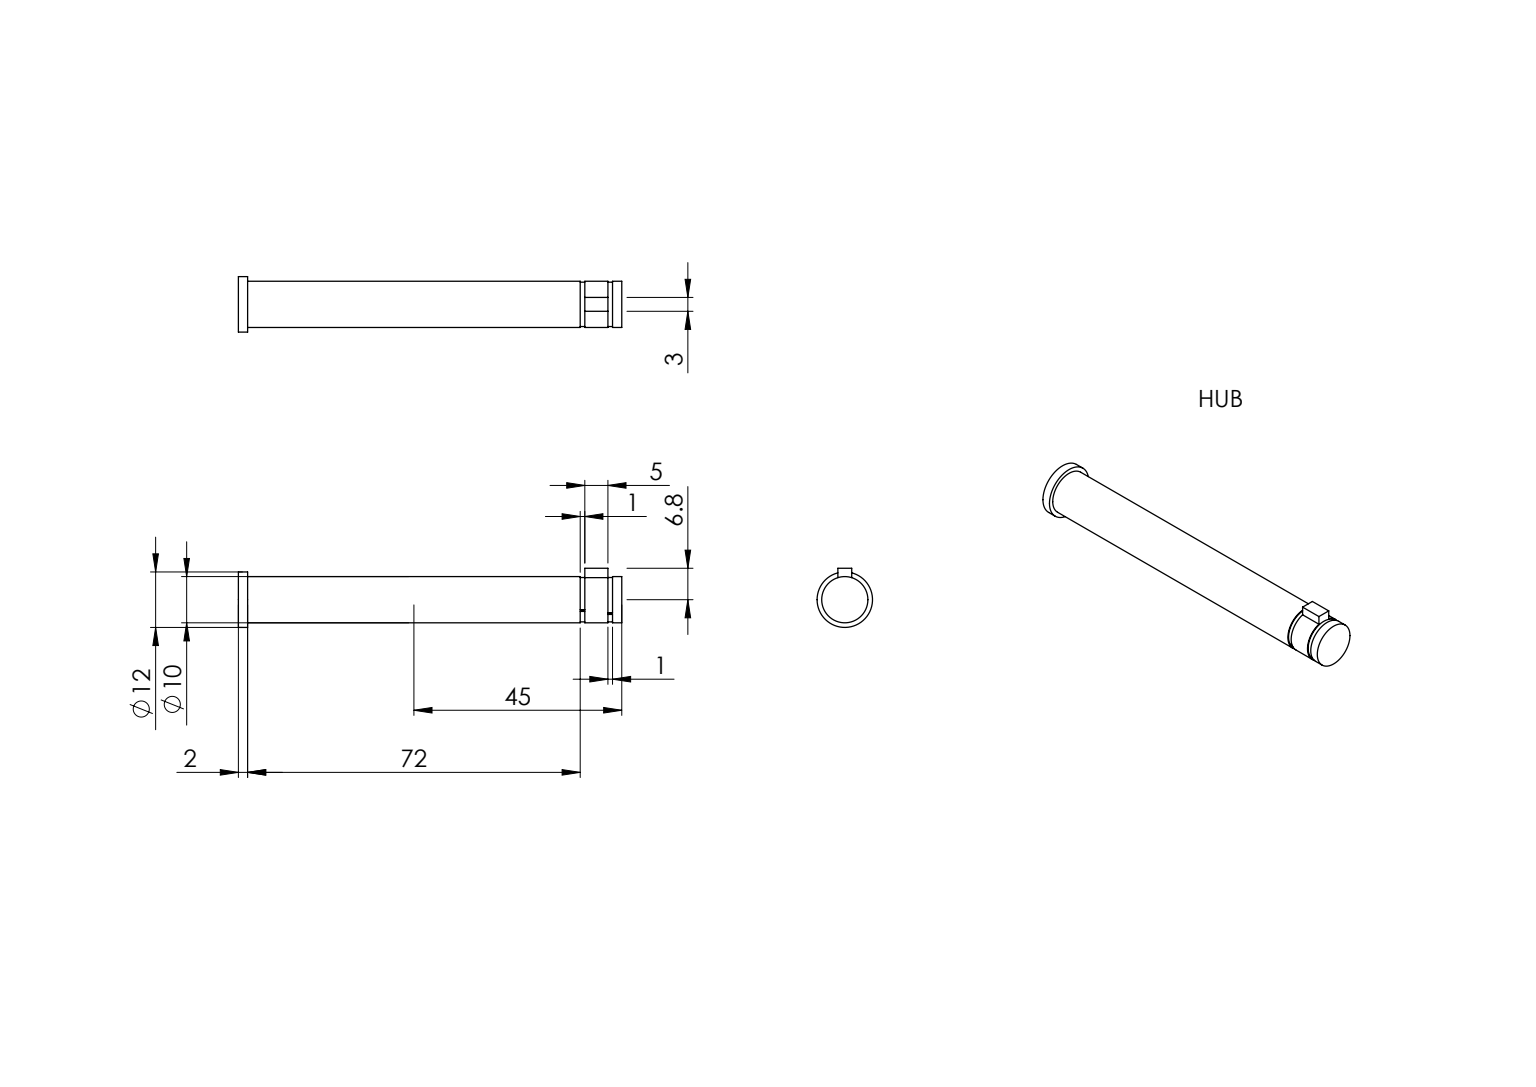
ISO-10303-21;
HEADER;
FILE_DESCRIPTION (('STEP AP214'),
    '1' );
FILE_NAME ('hub.step',
    '2026-10-27T08:02:39',
    ( '' ),
    ( '' ),
    'SwSTEP 2.0',
    'SolidWorks 2026',
    '' );
FILE_SCHEMA (( 'AUTOMOTIVE_DESIGN' ));
ENDSEC;

DATA;
#62=VECTOR ( 'NONE', #7382, 1000.000000000000000 ) ;
#68=DIRECTION ( 'NONE',  ( -1.000000000000000000, -3.903127820947815962E-18, 0.000000000000000000 ) ) ;
#73=CARTESIAN_POINT ( 'NONE',  ( 37.00000000000000711, 6.799999999999998046, 1.500000000000000000 ) ) ;
#88=VERTEX_POINT ( 'NONE', #10671 ) ;
#155=SHAPE_DEFINITION_REPRESENTATION ( #437, #678 ) ;
#172=VECTOR ( 'NONE', #10661, 1000.000000000000000 ) ;
#193=DIRECTION ( 'NONE',  ( -1.000000000000000000, -0.000000000000000000, -0.000000000000000000 ) ) ;
#207=DIRECTION ( 'NONE',  ( 1.000000000000000000, 0.000000000000000000, 0.000000000000000000 ) ) ;
#212=CARTESIAN_POINT ( 'NONE',  ( 0.000000000000000000, 0.000000000000000000, 0.000000000000000000 ) ) ;
#219=ADVANCED_FACE ( 'NONE', ( #2468 ), #6409, .F. ) ;
#236=DIRECTION ( 'NONE',  ( -1.000000000000000000, -3.903127820947815962E-18, 0.000000000000000000 ) ) ;
#259=MANIFOLD_SOLID_BREP ( 'Cavity1', #4172 ) ;
#260=CARTESIAN_POINT ( 'NONE',  ( -36.00000000000000000, 0.000000000000000000, 0.000000000000000000 ) ) ;
#285=EDGE_CURVE ( 'NONE', #11604, #9414, #8392, .T. ) ;
#314=DIRECTION ( 'NONE',  ( 0.000000000000000000, 0.000000000000000000, 1.000000000000000000 ) ) ;
#317=VERTEX_POINT ( 'NONE', #1844 ) ;
#319=DIRECTION ( 'NONE',  ( -1.000000000000000000, -0.000000000000000000, -0.000000000000000000 ) ) ;
#320=ORIENTED_EDGE ( 'NONE', *, *, #6145, .F. ) ;
#321=FACE_OUTER_BOUND ( 'NONE', #6866, .T. ) ;
#335=EDGE_LOOP ( 'NONE', ( #6954, #7348, #8380, #5572, #3850, #7690, #7602, #8198 ) ) ;
#344=VERTEX_POINT ( 'NONE', #10994 ) ;
#358=CYLINDRICAL_SURFACE ( 'NONE', #10659, 5.000000000000000000 ) ;
#371=CARTESIAN_POINT ( 'NONE',  ( 42.00000000000000000, 0.000000000000000000, 1.500000000000000000 ) ) ;
#436=CIRCLE ( 'NONE', #11425, 4.799999999999998934 ) ;
#437=PRODUCT_DEFINITION_SHAPE ( 'NONE', 'NONE',  #7937 ) ;
#448=LINE ( 'NONE', #6956, #1041 ) ;
#472=CARTESIAN_POINT ( 'NONE',  ( 37.00000000000000711, 0.000000000000000000, 0.000000000000000000 ) ) ;
#480=CARTESIAN_POINT ( 'NONE',  ( -38.00000000000000000, 0.000000000000000000, 0.000000000000000000 ) ) ;
#481=CARTESIAN_POINT ( 'NONE',  ( 43.00000000000000000, -3.792354139917827993, -2.942456469932580365 ) ) ;
#484=EDGE_CURVE ( 'NONE', #1854, #1927, #8266, .T. ) ;
#493=APPLICATION_CONTEXT ( 'automotive_design' ) ;
#502=EDGE_CURVE ( 'NONE', #1765, #8121, #3008, .T. ) ;
#503=EDGE_LOOP ( 'NONE', ( #1832, #534 ) ) ;
#504=VERTEX_POINT ( 'NONE', #4500 ) ;
#507=CYLINDRICAL_SURFACE ( 'NONE', #5435, 4.799999999999999822 ) ;
#512=ORIENTED_EDGE ( 'NONE', *, *, #3959, .T. ) ;
#514=PLANE ( 'NONE',  #6100 ) ;
#530=DIRECTION ( 'NONE',  ( 1.000000000000000000, 0.000000000000000000, 0.000000000000000000 ) ) ;
#534=ORIENTED_EDGE ( 'NONE', *, *, #8490, .T. ) ;
#539=ORIENTED_EDGE ( 'NONE', *, *, #11233, .F. ) ;
#551=CARTESIAN_POINT ( 'NONE',  ( 45.00000000000000000, 4.769696007084727185, 1.500000000000000000 ) ) ;
#595=EDGE_CURVE ( 'NONE', #3600, #7392, #2994, .T. ) ;
#609=CARTESIAN_POINT ( 'NONE',  ( 36.00000000000000711, -4.104405154062230115E-16, -2.224720805914714718E-17 ) ) ;
#646=CARTESIAN_POINT ( 'NONE',  ( 37.00000000000000711, -2.432816653220593039, 4.137801726981678030 ) ) ;
#655=AXIS2_PLACEMENT_3D ( 'NONE', #4690, #8568, #9509 ) ;
#662=EDGE_CURVE ( 'NONE', #5342, #3842, #7885, .T. ) ;
#669=AXIS2_PLACEMENT_3D ( 'NONE', #6757, #1749, #3818 ) ;
#678=SHAPE_REPRESENTATION ( 'hub', ( #6056 ), #8623 ) ;
#693=SURFACE_STYLE_FILL_AREA ( #10937 ) ;
#715=DIRECTION ( 'NONE',  ( 1.000000000000000000, 0.000000000000000000, 0.000000000000000000 ) ) ;
#731=ORIENTED_EDGE ( 'NONE', *, *, #5183, .F. ) ;
#733=VERTEX_POINT ( 'NONE', #6119 ) ;
#734=DIRECTION ( 'NONE',  ( 1.000000000000000000, -0.000000000000000000, 0.000000000000000000 ) ) ;
#748=FACE_OUTER_BOUND ( 'NONE', #2914, .T. ) ;
#762=VECTOR ( 'NONE', #7033, 1000.000000000000000 ) ;
#763=( NAMED_UNIT ( * ) SI_UNIT ( $, .STERADIAN. ) SOLID_ANGLE_UNIT ( ) );
#785=EDGE_CURVE ( 'NONE', #11661, #5342, #1300, .T. ) ;
#799=CARTESIAN_POINT ( 'NONE',  ( 42.00000000000000000, 6.799999999999998046, 1.500000000000000000 ) ) ;
#824=CARTESIAN_POINT ( 'NONE',  ( 43.00000000000000000, -2.824006678639516377, 3.881363971466655904 ) ) ;
#835=CARTESIAN_POINT ( 'NONE',  ( 42.00000000000000000, 0.000000000000000000, 0.000000000000000000 ) ) ;
#840=ADVANCED_FACE ( 'NONE', ( #2297 ), #10980, .F. ) ;
#846=CARTESIAN_POINT ( 'NONE',  ( 37.00000000000000711, -2.172883482918394282, 4.280020720704565740 ) ) ;
#856=ORIENTED_EDGE ( 'NONE', *, *, #10508, .F. ) ;
#914=EDGE_CURVE ( 'NONE', #4485, #1003, #11235, .T. ) ;
#920=LINE ( 'NONE', #10484, #4416 ) ;
#955=CARTESIAN_POINT ( 'NONE',  ( 45.00000000000000000, 0.000000000000000000, 0.000000000000000000 ) ) ;
#956=CARTESIAN_POINT ( 'NONE',  ( 37.00000000000000711, -4.104405154062230115E-16, -2.224720805914714718E-17 ) ) ;
#962=AXIS2_PLACEMENT_3D ( 'NONE', #956, #4845, #9481 ) ;
#973=ORIENTED_EDGE ( 'NONE', *, *, #8939, .F. ) ;
#1003=VERTEX_POINT ( 'NONE', #9431 ) ;
#1025=CYLINDRICAL_SURFACE ( 'NONE', #6817, 5.999999999999999112 ) ;
#1033=ORIENTED_EDGE ( 'NONE', *, *, #285, .T. ) ;
#1041=VECTOR ( 'NONE', #11748, 1000.000000000000000 ) ;
#1088=ORIENTED_EDGE ( 'NONE', *, *, #8797, .T. ) ;
#1115=DIRECTION ( 'NONE',  ( -1.000000000000000000, 0.000000000000000000, 0.000000000000000000 ) ) ;
#1116=EDGE_CURVE ( 'NONE', #5049, #6113, #10419, .T. ) ;
#1122=DIRECTION ( 'NONE',  ( 0.000000000000000000, 0.000000000000000000, 1.000000000000000000 ) ) ;
#1172=CIRCLE ( 'NONE', #4361, 5.000000000000000000 ) ;
#1191=ADVANCED_FACE ( 'NONE', ( #5103 ), #5223, .F. ) ;
#1199=VECTOR ( 'NONE', #1553, 1000.000000000000000 ) ;
#1211=CARTESIAN_POINT ( 'NONE',  ( 45.00000000000000000, 6.123233995736765296E-16, -5.000000000000000000 ) ) ;
#1224=AXIS2_PLACEMENT_3D ( 'NONE', #1581, #3763, #11268 ) ;
#1228=AXIS2_PLACEMENT_3D ( 'NONE', #480, #7310, #3543 ) ;
#1247=ORIENTED_EDGE ( 'NONE', *, *, #1673, .T. ) ;
#1270=VERTEX_POINT ( 'NONE', #4974 ) ;
#1287=DIRECTION ( 'NONE',  ( 0.000000000000000000, 0.8620420264545162192, 0.5068368027542899945 ) ) ;
#1300=LINE ( 'NONE', #3182, #1608 ) ;
#1353=ADVANCED_FACE ( 'NONE', ( #8293 ), #12082, .T. ) ;
#1370=CARTESIAN_POINT ( 'NONE',  ( 36.00000000000000711, 4.210917358895616580, 2.303947698310782943 ) ) ;
#1375=PLANE ( 'NONE',  #5221 ) ;
#1378=DIRECTION ( 'NONE',  ( 0.000000000000000000, 0.8772744497699203059, 0.4799891038147465760 ) ) ;
#1381=ORIENTED_EDGE ( 'NONE', *, *, #5937, .F. ) ;
#1410=ORIENTED_EDGE ( 'NONE', *, *, #6663, .T. ) ;
#1415=CARTESIAN_POINT ( 'NONE',  ( 37.00000000000000711, 0.000000000000000000, 0.000000000000000000 ) ) ;
#1422=AXIS2_PLACEMENT_3D ( 'NONE', #4926, #236, #11538 ) ;
#1452=( NAMED_UNIT ( * ) PLANE_ANGLE_UNIT ( ) SI_UNIT ( $, .RADIAN. ) );
#1458=ADVANCED_FACE ( 'NONE', ( #2845 ), #8721, .T. ) ;
#1465=CARTESIAN_POINT ( 'NONE',  ( 36.00000000000000711, 6.123233995736765296E-16, -5.000000000000000000 ) ) ;
#1495=ORIENTED_EDGE ( 'NONE', *, *, #595, .F. ) ;
#1503=DIRECTION ( 'NONE',  ( 1.301452268327822979E-17, 0.7707772616747329275, 0.6371047110838219396 ) ) ;
#1507=ORIENTED_EDGE ( 'NONE', *, *, #10328, .T. ) ;
#1510=( NAMED_UNIT ( * ) SI_UNIT ( $, .STERADIAN. ) SOLID_ANGLE_UNIT ( ) );
#1536=EDGE_CURVE ( 'NONE', #5049, #317, #11146, .T. ) ;
#1546=CARTESIAN_POINT ( 'NONE',  ( 43.00000000000000000, 3.903127820947864496E-18, 0.000000000000000000 ) ) ;
#1549=PLANE ( 'NONE',  #4101 ) ;
#1553=DIRECTION ( 'NONE',  ( 1.000000000000000000, -0.000000000000000000, -0.000000000000000000 ) ) ;
#1562=( LENGTH_UNIT ( ) NAMED_UNIT ( * ) SI_UNIT ( .MILLI., .METRE. ) );
#1577=VECTOR ( 'NONE', #9990, 1000.000000000000000 ) ;
#1581=CARTESIAN_POINT ( 'NONE',  ( 37.00000000000000711, 0.000000000000000000, 0.000000000000000000 ) ) ;
#1582=ORIENTED_EDGE ( 'NONE', *, *, #11605, .T. ) ;
#1608=VECTOR ( 'NONE', #3129, 1000.000000000000000 ) ;
#1610=DIRECTION ( 'NONE',  ( -1.000000000000000000, -0.000000000000000000, -0.000000000000000000 ) ) ;
#1611=ORIENTED_EDGE ( 'NONE', *, *, #8738, .F. ) ;
#1621=AXIS2_PLACEMENT_3D ( 'NONE', #10075, #1503, #9432 ) ;
#1627=ORIENTED_EDGE ( 'NONE', *, *, #12236, .T. ) ;
#1628=ORIENTED_EDGE ( 'NONE', *, *, #11881, .F. ) ;
#1629=EDGE_CURVE ( 'NONE', #1765, #8354, #6857, .T. ) ;
#1660=CIRCLE ( 'NONE', #11831, 4.799999999999998934 ) ;
#1661=CARTESIAN_POINT ( 'NONE',  ( 29.56763832957518545, 0.000000000000000000, -1.500000000000000000 ) ) ;
#1664=CARTESIAN_POINT ( 'NONE',  ( 42.00000000000000000, -3.185523555419110586, 3.853886308373666747 ) ) ;
#1673=EDGE_CURVE ( 'NONE', #317, #10112, #11885, .T. ) ;
#1678=EDGE_LOOP ( 'NONE', ( #10121, #11349, #11716, #1582 ) ) ;
#1682=ORIENTED_EDGE ( 'NONE', *, *, #5930, .F. ) ;
#1689=CARTESIAN_POINT ( 'NONE',  ( 42.00000000000000000, 0.000000000000000000, 0.000000000000000000 ) ) ;
#1695=CARTESIAN_POINT ( 'NONE',  ( 37.00000000000000711, 4.769696007084728073, 1.500000000000000444 ) ) ;
#1727=CARTESIAN_POINT ( 'NONE',  ( 36.00000000000000711, -4.210917358895616580, -2.303947698310783387 ) ) ;
#1749=DIRECTION ( 'NONE',  ( -1.000000000000000000, 0.000000000000000000, 0.000000000000000000 ) ) ;
#1765=VERTEX_POINT ( 'NONE', #1465 ) ;
#1774=CARTESIAN_POINT ( 'NONE',  ( 37.00000000000000711, -4.104405154062230115E-16, -2.224720805914714718E-17 ) ) ;
#1804=EDGE_CURVE ( 'NONE', #1003, #10175, #6281, .T. ) ;
#1816=CARTESIAN_POINT ( 'NONE',  ( 42.00000000000000000, 0.000000000000000000, 5.000000000000000000 ) ) ;
#1826=AXIS2_PLACEMENT_3D ( 'NONE', #4983, #1115, #8885 ) ;
#1832=ORIENTED_EDGE ( 'NONE', *, *, #7750, .T. ) ;
#1844=CARTESIAN_POINT ( 'NONE',  ( 37.00000000000000711, 4.210917358895616580, 2.303947698310782943 ) ) ;
#1848=CARTESIAN_POINT ( 'NONE',  ( -38.00000000000000000, 0.000000000000000000, 0.000000000000000000 ) ) ;
#1854=VERTEX_POINT ( 'NONE', #2566 ) ;
#1864=ORIENTED_EDGE ( 'NONE', *, *, #7519, .T. ) ;
#1866=CARTESIAN_POINT ( 'NONE',  ( 37.00000000000000711, -4.210917358895617468, -2.303947698310783831 ) ) ;
#1868=DIRECTION ( 'NONE',  ( -1.000000000000000000, -0.000000000000000000, -0.000000000000000000 ) ) ;
#1880=ADVANCED_FACE ( 'NONE', ( #10029 ), #514, .T. ) ;
#1890=VERTEX_POINT ( 'NONE', #5462 ) ;
#1893=CARTESIAN_POINT ( 'NONE',  ( -38.00000000000000000, 0.000000000000000000, 0.000000000000000000 ) ) ;
#1901=CARTESIAN_POINT ( 'NONE',  ( 45.00000000000000000, 0.000000000000000000, 0.000000000000000000 ) ) ;
#1920=UNCERTAINTY_MEASURE_WITH_UNIT (LENGTH_MEASURE( 1.000000000000000082E-05 ), #4525, 'distance_accuracy_value', 'NONE');
#1927=VERTEX_POINT ( 'NONE', #12308 ) ;
#1936=LINE ( 'NONE', #7695, #2299 ) ;
#1984=DIRECTION ( 'NONE',  ( -1.000000000000000000, 0.000000000000000000, 0.000000000000000000 ) ) ;
#1999=DIRECTION ( 'NONE',  ( 1.000000000000000000, 0.000000000000000000, 0.000000000000000000 ) ) ;
#2001=FACE_OUTER_BOUND ( 'NONE', #2830, .T. ) ;
#2018=PLANE ( 'NONE',  #4439 ) ;
#2035=AXIS2_PLACEMENT_3D ( 'NONE', #1901, #319, #4136 ) ;
#2064=CARTESIAN_POINT ( 'NONE',  ( 29.56763832957518545, 6.799999999999998046, 1.500000000000000000 ) ) ;
#2069=CARTESIAN_POINT ( 'NONE',  ( -38.00000000000000000, 0.000000000000000000, 0.000000000000000000 ) ) ;
#2089=AXIS2_PLACEMENT_3D ( 'NONE', #2200, #6087, #4262 ) ;
#2097=VERTEX_POINT ( 'NONE', #5007 ) ;
#2112=ORIENTED_EDGE ( 'NONE', *, *, #7381, .T. ) ;
#2127=LINE ( 'NONE', #3998, #2490 ) ;
#2131=EDGE_CURVE ( 'NONE', #7392, #1890, #2203, .T. ) ;
#2139=CYLINDRICAL_SURFACE ( 'NONE', #2089, 4.799999999999998934 ) ;
#2200=CARTESIAN_POINT ( 'NONE',  ( 43.00000000000000000, 3.903127820947864496E-18, 0.000000000000000000 ) ) ;
#2201=ORIENTED_EDGE ( 'NONE', *, *, #9315, .T. ) ;
#2203=CIRCLE ( 'NONE', #3012, 5.000000000000000000 ) ;
#2204=AXIS2_PLACEMENT_3D ( 'NONE', #9934, #7123, #9993 ) ;
#2206=CARTESIAN_POINT ( 'NONE',  ( 37.00000000000000711, 4.210917358895617468, 2.303947698310783387 ) ) ;
#2213=ORIENTED_EDGE ( 'NONE', *, *, #4563, .T. ) ;
#2266=LINE ( 'NONE', #11006, #9628 ) ;
#2295=CARTESIAN_POINT ( 'NONE',  ( 37.00000000000000711, 0.000000000000000000, 5.000000000000000000 ) ) ;
#2297=FACE_OUTER_BOUND ( 'NONE', #12132, .T. ) ;
#2299=VECTOR ( 'NONE', #2930, 1000.000000000000114 ) ;
#2305=ORIENTED_EDGE ( 'NONE', *, *, #12265, .T. ) ;
#2313=ORIENTED_EDGE ( 'NONE', *, *, #12104, .T. ) ;
#2348=FACE_OUTER_BOUND ( 'NONE', #9404, .T. ) ;
#2349=LINE ( 'NONE', #481, #1577 ) ;
#2373=CARTESIAN_POINT ( 'NONE',  ( 42.00000000000000000, 0.000000000000000000, 0.000000000000000000 ) ) ;
#2378=VECTOR ( 'NONE', #7623, 1000.000000000000000 ) ;
#2399=EDGE_CURVE ( 'NONE', #11586, #6059, #3867, .T. ) ;
#2413=LINE ( 'NONE', #9178, #11991 ) ;
#2423=ORIENTED_EDGE ( 'NONE', *, *, #662, .F. ) ;
#2438=FACE_OUTER_BOUND ( 'NONE', #9609, .T. ) ;
#2451=CIRCLE ( 'NONE', #655, 5.000000000000000000 ) ;
#2453=CARTESIAN_POINT ( 'NONE',  ( 43.00000000000000000, 3.792354139917828437, 2.942456469932579921 ) ) ;
#2456=CARTESIAN_POINT ( 'NONE',  ( 29.56763832957518545, 6.799999999999998046, -1.500000000000000000 ) ) ;
#2468=FACE_OUTER_BOUND ( 'NONE', #11107, .T. ) ;
#2490=VECTOR ( 'NONE', #5178, 1000.000000000000000 ) ;
#2506=CARTESIAN_POINT ( 'NONE',  ( 42.00000000000000000, 4.814824860968089633E-32, 0.000000000000000000 ) ) ;
#2515=VERTEX_POINT ( 'NONE', #6161 ) ;
#2521=UNCERTAINTY_MEASURE_WITH_UNIT (LENGTH_MEASURE( 1.000000000000000082E-05 ), #1562, 'distance_accuracy_value', 'NONE');
#2523=DIRECTION ( 'NONE',  ( -0.000000000000000000, 0.000000000000000000, 1.000000000000000000 ) ) ;
#2566=CARTESIAN_POINT ( 'NONE',  ( -38.00000000000000000, 7.347880794884118750E-16, 5.999999999999999112 ) ) ;
#2604=LINE ( 'NONE', #11168, #7784 ) ;
#2620=DIRECTION ( 'NONE',  ( 0.000000000000000000, -0.000000000000000000, 1.000000000000000000 ) ) ;
#2639=ORIENTED_EDGE ( 'NONE', *, *, #12100, .T. ) ;
#2643=ORIENTED_EDGE ( 'NONE', *, *, #10890, .T. ) ;
#2649=ORIENTED_EDGE ( 'NONE', *, *, #2131, .F. ) ;
#2682=ORIENTED_EDGE ( 'NONE', *, *, #8074, .T. ) ;
#2704=CYLINDRICAL_SURFACE ( 'NONE', #10959, 5.000000000000000000 ) ;
#2757=DIRECTION ( 'NONE',  ( -1.000000000000000000, -0.000000000000000000, -0.000000000000000000 ) ) ;
#2788=ADVANCED_FACE ( 'NONE', ( #4960 ), #11330, .T. ) ;
#2810=DIRECTION ( 'NONE',  ( 1.000000000000000000, 3.903127820947815962E-18, 0.000000000000000000 ) ) ;
#2813=CARTESIAN_POINT ( 'NONE',  ( 37.00000000000000711, -2.172883482918394282, 4.280020720704565740 ) ) ;
#2823=CIRCLE ( 'NONE', #1224, 5.000000000000000000 ) ;
#2830=EDGE_LOOP ( 'NONE', ( #3983, #4790 ) ) ;
#2840=AXIS2_PLACEMENT_3D ( 'NONE', #3637, #11258, #6515 ) ;
#2845=FACE_OUTER_BOUND ( 'NONE', #1678, .T. ) ;
#2850=ORIENTED_EDGE ( 'NONE', *, *, #5097, .F. ) ;
#2899=EDGE_LOOP ( 'NONE', ( #10933, #2313, #4925, #5764 ) ) ;
#2906=DIRECTION ( 'NONE',  ( 0.000000000000000000, -1.000000000000000000, 0.000000000000000000 ) ) ;
#2914=EDGE_LOOP ( 'NONE', ( #7933, #4511, #5973, #1682, #1410, #12158, #11727, #539, #8955, #3912, #4287, #6695, #5729, #6234, #10391, #6437, #8922, #1033, #4967, #731 ) ) ;
#2925=ORIENTED_EDGE ( 'NONE', *, *, #10981, .F. ) ;
#2926=DIRECTION ( 'NONE',  ( 0.000000000000000000, 0.7900737791495477946, 0.6130117645692876316 ) ) ;
#2929=ORIENTED_EDGE ( 'NONE', *, *, #785, .F. ) ;
#2930=DIRECTION ( 'NONE',  ( 2.817067928751547788E-17, 0.6371047110838219396, -0.7707772616747329275 ) ) ;
#2944=EDGE_CURVE ( 'NONE', #1270, #4573, #7150, .T. ) ;
#2980=CARTESIAN_POINT ( 'NONE',  ( 45.00000000000000000, 0.000000000000000000, 5.000000000000000000 ) ) ;
#2994=LINE ( 'NONE', #10496, #5001 ) ;
#2996=VERTEX_POINT ( 'NONE', #10847 ) ;
#3006=ORIENTED_EDGE ( 'NONE', *, *, #3674, .F. ) ;
#3008=CIRCLE ( 'NONE', #7008, 5.000000000000000000 ) ;
#3012=AXIS2_PLACEMENT_3D ( 'NONE', #4006, #11690, #314 ) ;
#3031=DIRECTION ( 'NONE',  ( 1.000000000000000000, -0.000000000000000000, -0.000000000000000000 ) ) ;
#3053=LINE ( 'NONE', #8610, #4796 ) ;
#3068=FACE_BOUND ( 'NONE', #7491, .T. ) ;
#3074=ORIENTED_EDGE ( 'NONE', *, *, #11605, .F. ) ;
#3117=EDGE_CURVE ( 'NONE', #2097, #8354, #3445, .T. ) ;
#3129=DIRECTION ( 'NONE',  ( 0.000000000000000000, 1.000000000000000000, -0.000000000000000000 ) ) ;
#3147=ORIENTED_EDGE ( 'NONE', *, *, #5391, .F. ) ;
#3151=FACE_OUTER_BOUND ( 'NONE', #3282, .T. ) ;
#3182=CARTESIAN_POINT ( 'NONE',  ( 37.00000000000000711, 0.000000000000000000, 1.500000000000000000 ) ) ;
#3188=CARTESIAN_POINT ( 'NONE',  ( 43.00000000000000000, -3.058102613202345665, 3.699730856038719207 ) ) ;
#3193=VERTEX_POINT ( 'NONE', #7288 ) ;
#3201=CARTESIAN_POINT ( 'NONE',  ( 42.00000000000000000, 6.799999999999998046, -1.500000000000000000 ) ) ;
#3218=CARTESIAN_POINT ( 'NONE',  ( 45.00000000000000000, 6.123233995736765296E-16, -5.000000000000000000 ) ) ;
#3222=AXIS2_PLACEMENT_3D ( 'NONE', #1893, #3757, #4943 ) ;
#3223=ORIENTED_EDGE ( 'NONE', *, *, #9680, .T. ) ;
#3262=ORIENTED_EDGE ( 'NONE', *, *, #7381, .F. ) ;
#3263=DIRECTION ( 'NONE',  ( -1.000000000000000000, -0.000000000000000000, -0.000000000000000000 ) ) ;
#3274=ADVANCED_FACE ( 'NONE', ( #10571 ), #2018, .F. ) ;
#3282=EDGE_LOOP ( 'NONE', ( #9061, #8705, #2213, #3750 ) ) ;
#3300=DIRECTION ( 'NONE',  ( 0.000000000000000000, 0.000000000000000000, -1.000000000000000000 ) ) ;
#3303=CARTESIAN_POINT ( 'NONE',  ( 42.00000000000000000, 0.000000000000000000, 0.000000000000000000 ) ) ;
#3307=CYLINDRICAL_SURFACE ( 'NONE', #1228, 5.999999999999999112 ) ;
#3342=DIRECTION ( 'NONE',  ( 0.000000000000000000, 0.5068368027542901055, -0.8620420264545163302 ) ) ;
#3348=FACE_OUTER_BOUND ( 'NONE', #7452, .T. ) ;
#3369=VECTOR ( 'NONE', #8356, 1000.000000000000000 ) ;
#3384=EDGE_LOOP ( 'NONE', ( #6916, #11579, #5274, #3074, #7548, #5520, #3726, #2649 ) ) ;
#3445=CIRCLE ( 'NONE', #6654, 5.000000000000000000 ) ;
#3458=VECTOR ( 'NONE', #12276, 1000.000000000000000 ) ;
#3464=AXIS2_PLACEMENT_3D ( 'NONE', #9092, #8273, #9143 ) ;
#3483=CIRCLE ( 'NONE', #7884, 4.799999999999999822 ) ;
#3523=CARTESIAN_POINT ( 'NONE',  ( -36.00000000000000000, 0.000000000000000000, 0.000000000000000000 ) ) ;
#3525=CARTESIAN_POINT ( 'NONE',  ( 42.00000000000000000, -3.058102613202345665, 3.699730856038719207 ) ) ;
#3532=DIRECTION ( 'NONE',  ( -1.000000000000000000, -3.903127820947815962E-18, 0.000000000000000000 ) ) ;
#3543=DIRECTION ( 'NONE',  ( 0.000000000000000000, 0.000000000000000000, -1.000000000000000000 ) ) ;
#3561=LINE ( 'NONE', #551, #62 ) ;
#3583=AXIS2_PLACEMENT_3D ( 'NONE', #1546, #5362, #2926 ) ;
#3600=VERTEX_POINT ( 'NONE', #11919 ) ;
#3628=CIRCLE ( 'NONE', #8235, 5.999999999999999112 ) ;
#3637=CARTESIAN_POINT ( 'NONE',  ( 45.00000000000000000, 0.000000000000000000, 0.000000000000000000 ) ) ;
#3656=EDGE_LOOP ( 'NONE', ( #10124, #9210, #8933, #10573 ) ) ;
#3658=UNCERTAINTY_MEASURE_WITH_UNIT (LENGTH_MEASURE( 1.000000000000000082E-05 ), #4312, 'distance_accuracy_value', 'NONE');
#3666=VERTEX_POINT ( 'NONE', #4366 ) ;
#3668=DIRECTION ( 'NONE',  ( 0.000000000000000000, -0.4526840589413320126, 0.8916709834801178625 ) ) ;
#3674=EDGE_CURVE ( 'NONE', #733, #4573, #2451, .T. ) ;
#3699=EDGE_CURVE ( 'NONE', #11604, #504, #7641, .T. ) ;
#3726=ORIENTED_EDGE ( 'NONE', *, *, #9315, .F. ) ;
#3750=ORIENTED_EDGE ( 'NONE', *, *, #1673, .F. ) ;
#3757=DIRECTION ( 'NONE',  ( -1.000000000000000000, 0.000000000000000000, 0.000000000000000000 ) ) ;
#3762=DIRECTION ( 'NONE',  ( 1.000000000000000000, 0.000000000000000000, 0.000000000000000000 ) ) ;
#3763=DIRECTION ( 'NONE',  ( -1.000000000000000000, 0.000000000000000000, 0.000000000000000000 ) ) ;
#3796=EDGE_CURVE ( 'NONE', #10109, #88, #4880, .T. ) ;
#3818=DIRECTION ( 'NONE',  ( 0.000000000000000000, 0.000000000000000000, 1.000000000000000000 ) ) ;
#3842=VERTEX_POINT ( 'NONE', #799 ) ;
#3850=ORIENTED_EDGE ( 'NONE', *, *, #10825, .T. ) ;
#3867=LINE ( 'NONE', #2980, #7824 ) ;
#3906=AXIS2_PLACEMENT_3D ( 'NONE', #10256, #5513, #7281 ) ;
#3912=ORIENTED_EDGE ( 'NONE', *, *, #2131, .T. ) ;
#3942=DIRECTION ( 'NONE',  ( 1.000000000000000000, 3.903127820947815962E-18, 0.000000000000000000 ) ) ;
#3955=ORIENTED_EDGE ( 'NONE', *, *, #7519, .F. ) ;
#3959=EDGE_CURVE ( 'NONE', #4240, #3193, #4659, .T. ) ;
#3962=LINE ( 'NONE', #8105, #8230 ) ;
#3970=PRODUCT_CONTEXT ( 'NONE', #7938, 'mechanical' ) ;
#3983=ORIENTED_EDGE ( 'NONE', *, *, #8738, .T. ) ;
#3987=FACE_OUTER_BOUND ( 'NONE', #3656, .T. ) ;
#3998=CARTESIAN_POINT ( 'NONE',  ( 42.00000000000000000, 6.799999999999998046, 0.000000000000000000 ) ) ;
#4006=CARTESIAN_POINT ( 'NONE',  ( 36.00000000000000711, 0.000000000000000000, 0.000000000000000000 ) ) ;
#4015=CYLINDRICAL_SURFACE ( 'NONE', #11066, 4.799999999999999822 ) ;
#4018=CARTESIAN_POINT ( 'NONE',  ( 42.00000000000000000, 0.000000000000000000, -1.500000000000000000 ) ) ;
#4028=STYLED_ITEM ( 'NONE', ( #4507 ), #9458 ) ;
#4035=DIRECTION ( 'NONE',  ( 0.000000000000000000, 0.000000000000000000, 1.000000000000000000 ) ) ;
#4073=DIRECTION ( 'NONE',  ( 0.000000000000000000, 0.000000000000000000, 1.000000000000000000 ) ) ;
#4101=AXIS2_PLACEMENT_3D ( 'NONE', #609, #12101, #7373 ) ;
#4117=EDGE_CURVE ( 'NONE', #7407, #1927, #6063, .T. ) ;
#4136=DIRECTION ( 'NONE',  ( 0.000000000000000000, 0.000000000000000000, 1.000000000000000000 ) ) ;
#4155=CARTESIAN_POINT ( 'NONE',  ( 36.00000000000000711, 0.000000000000000000, 0.000000000000000000 ) ) ;
#4158=DIRECTION ( 'NONE',  ( 0.000000000000000000, 0.8772744497699203059, 0.4799891038147465760 ) ) ;
#4162=DIRECTION ( 'NONE',  ( -1.000000000000000000, -3.903127820947815962E-18, 0.000000000000000000 ) ) ;
#4166=EDGE_CURVE ( 'NONE', #3193, #88, #1660, .T. ) ;
#4172=CLOSED_SHELL ( 'NONE', ( #5078, #11502, #5002, #8330, #5958, #4295, #7700, #10074, #6499, #11433, #1353, #8462, #10468, #5865, #219, #2788, #11453, #10216, #9282, #8997, #3274, #1880, #5871, #1191, #840, #5612, #1458 ) ) ;
#4176=DIRECTION ( 'NONE',  ( -1.000000000000000000, -3.903127820947815962E-18, 0.000000000000000000 ) ) ;
#4211=EDGE_LOOP ( 'NONE', ( #7282, #5737, #10480, #8162 ) ) ;
#4240=VERTEX_POINT ( 'NONE', #6708 ) ;
#4256=VERTEX_POINT ( 'NONE', #10635 ) ;
#4262=DIRECTION ( 'NONE',  ( 0.000000000000000000, 0.7900737791495477946, 0.6130117645692876316 ) ) ;
#4270=EDGE_CURVE ( 'NONE', #9277, #7555, #5943, .T. ) ;
#4274=DIRECTION ( 'NONE',  ( 0.000000000000000000, 0.000000000000000000, -1.000000000000000000 ) ) ;
#4287=ORIENTED_EDGE ( 'NONE', *, *, #11100, .T. ) ;
#4293=ORIENTED_EDGE ( 'NONE', *, *, #11723, .F. ) ;
#4295=ADVANCED_FACE ( 'NONE', ( #5891 ), #358, .T. ) ;
#4312=( LENGTH_UNIT ( ) NAMED_UNIT ( * ) SI_UNIT ( .MILLI., .METRE. ) );
#4361=AXIS2_PLACEMENT_3D ( 'NONE', #1415, #5240, #6244 ) ;
#4366=CARTESIAN_POINT ( 'NONE',  ( 43.00000000000000000, -2.941673623582830022, 4.043087470277766826 ) ) ;
#4383=CARTESIAN_POINT ( 'NONE',  ( 43.00000000000000000, 3.903127820947864496E-18, 0.000000000000000000 ) ) ;
#4392=DIRECTION ( 'NONE',  ( 1.000000000000000000, 3.903127820947815962E-18, 0.000000000000000000 ) ) ;
#4409=AXIS2_PLACEMENT_3D ( 'NONE', #5979, #1287, #8983 ) ;
#4416=VECTOR ( 'NONE', #10420, 1000.000000000000114 ) ;
#4439=AXIS2_PLACEMENT_3D ( 'NONE', #824, #7769, #7581 ) ;
#4446=( NAMED_UNIT ( * ) PLANE_ANGLE_UNIT ( ) SI_UNIT ( $, .RADIAN. ) );
#4481=CARTESIAN_POINT ( 'NONE',  ( 37.00000000000000711, 0.000000000000000000, 0.000000000000000000 ) ) ;
#4485=VERTEX_POINT ( 'NONE', #12333 ) ;
#4500=CARTESIAN_POINT ( 'NONE',  ( 37.00000000000000711, 6.123233995736765296E-16, -5.000000000000000000 ) ) ;
#4507=PRESENTATION_STYLE_ASSIGNMENT (( #11072 ) ) ;
#4511=ORIENTED_EDGE ( 'NONE', *, *, #7750, .F. ) ;
#4525=( LENGTH_UNIT ( ) NAMED_UNIT ( * ) SI_UNIT ( .MILLI., .METRE. ) );
#4526=FACE_OUTER_BOUND ( 'NONE', #9415, .T. ) ;
#4527=DIRECTION ( 'NONE',  ( 0.000000000000000000, 0.000000000000000000, -1.000000000000000000 ) ) ;
#4531=ORIENTED_EDGE ( 'NONE', *, *, #10127, .T. ) ;
#4540=CARTESIAN_POINT ( 'NONE',  ( 37.00000000000000711, -2.432816653220593039, 4.137801726981678030 ) ) ;
#4543=ORIENTED_EDGE ( 'NONE', *, *, #484, .F. ) ;
#4549=DIRECTION ( 'NONE',  ( 0.000000000000000000, 0.8772744497699203059, 0.4799891038147465760 ) ) ;
#4554=EDGE_CURVE ( 'NONE', #344, #11586, #8887, .T. ) ;
#4563=EDGE_CURVE ( 'NONE', #6113, #10112, #3483, .T. ) ;
#4573=VERTEX_POINT ( 'NONE', #6153 ) ;
#4578=ORIENTED_EDGE ( 'NONE', *, *, #1629, .T. ) ;
#4623=AXIS2_PLACEMENT_3D ( 'NONE', #10104, #715, #4527 ) ;
#4635=ORIENTED_EDGE ( 'NONE', *, *, #10732, .F. ) ;
#4659=CIRCLE ( 'NONE', #3464, 4.799999999999998934 ) ;
#4662=CYLINDRICAL_SURFACE ( 'NONE', #7193, 4.799999999999998934 ) ;
#4690=CARTESIAN_POINT ( 'NONE',  ( 43.00000000000000000, 0.000000000000000000, 0.000000000000000000 ) ) ;
#4713=EDGE_CURVE ( 'NONE', #10072, #6450, #6477, .T. ) ;
#4737=ORIENTED_EDGE ( 'NONE', *, *, #5956, .T. ) ;
#4740=ORIENTED_EDGE ( 'NONE', *, *, #8490, .F. ) ;
#4746=DIRECTION ( 'NONE',  ( -1.000000000000000000, -0.000000000000000000, -0.000000000000000000 ) ) ;
#4790=ORIENTED_EDGE ( 'NONE', *, *, #5097, .T. ) ;
#4796=VECTOR ( 'NONE', #11473, 1000.000000000000000 ) ;
#4845=DIRECTION ( 'NONE',  ( 1.000000000000000000, -0.000000000000000000, 0.000000000000000000 ) ) ;
#4854=VERTEX_POINT ( 'NONE', #9662 ) ;
#4880=LINE ( 'NONE', #8700, #10836 ) ;
#4895=DIRECTION ( 'NONE',  ( 0.000000000000000000, 0.000000000000000000, 1.000000000000000000 ) ) ;
#4925=ORIENTED_EDGE ( 'NONE', *, *, #10277, .T. ) ;
#4926=CARTESIAN_POINT ( 'NONE',  ( 43.00000000000000000, 3.903127820947864496E-18, 0.000000000000000000 ) ) ;
#4943=DIRECTION ( 'NONE',  ( 0.000000000000000000, 0.000000000000000000, 1.000000000000000000 ) ) ;
#4946=CYLINDRICAL_SURFACE ( 'NONE', #8256, 5.000000000000000000 ) ;
#4954=DIRECTION ( 'NONE',  ( 0.000000000000000000, 0.000000000000000000, 1.000000000000000000 ) ) ;
#4960=FACE_OUTER_BOUND ( 'NONE', #7354, .T. ) ;
#4967=ORIENTED_EDGE ( 'NONE', *, *, #5306, .T. ) ;
#4974=CARTESIAN_POINT ( 'NONE',  ( 45.00000000000000000, 6.123233995736765296E-16, -5.000000000000000000 ) ) ;
#4983=CARTESIAN_POINT ( 'NONE',  ( -36.00000000000000000, 0.000000000000000000, 0.000000000000000000 ) ) ;
#4993=ORIENTED_EDGE ( 'NONE', *, *, #10277, .F. ) ;
#4994=DIRECTION ( 'NONE',  ( 0.000000000000000000, 0.000000000000000000, 1.000000000000000000 ) ) ;
#5001=VECTOR ( 'NONE', #7751, 1000.000000000000000 ) ;
#5002=ADVANCED_FACE ( 'NONE', ( #321 ), #2139, .T. ) ;
#5007=CARTESIAN_POINT ( 'NONE',  ( -36.00000000000000000, 0.000000000000000000, 5.000000000000000000 ) ) ;
#5049=VERTEX_POINT ( 'NONE', #10709 ) ;
#5051=AXIS2_PLACEMENT_3D ( 'NONE', #10882, #6131, #2620 ) ;
#5057=CARTESIAN_POINT ( 'NONE',  ( 43.00000000000000000, 0.000000000000000000, 0.000000000000000000 ) ) ;
#5075=PLANE ( 'NONE',  #5051 ) ;
#5078=ADVANCED_FACE ( 'NONE', ( #3151 ), #4015, .T. ) ;
#5080=FACE_OUTER_BOUND ( 'NONE', #8186, .T. ) ;
#5094=CARTESIAN_POINT ( 'NONE',  ( 42.00000000000000000, 0.000000000000000000, 0.000000000000000000 ) ) ;
#5097=EDGE_CURVE ( 'NONE', #1854, #9966, #5288, .T. ) ;
#5103=FACE_OUTER_BOUND ( 'NONE', #7406, .T. ) ;
#5123=CARTESIAN_POINT ( 'NONE',  ( 45.00000000000000000, -2.941673623582828245, 4.043087470277764162 ) ) ;
#5131=VERTEX_POINT ( 'NONE', #10138 ) ;
#5167=AXIS2_PLACEMENT_3D ( 'NONE', #1689, #9381, #12058 ) ;
#5178=DIRECTION ( 'NONE',  ( 0.000000000000000000, 0.000000000000000000, 1.000000000000000000 ) ) ;
#5183=EDGE_CURVE ( 'NONE', #4573, #2515, #8898, .T. ) ;
#5216=VECTOR ( 'NONE', #10411, 1000.000000000000000 ) ;
#5220=AXIS2_PLACEMENT_3D ( 'NONE', #472, #530, #3300 ) ;
#5221=AXIS2_PLACEMENT_3D ( 'NONE', #2373, #5326, #10084 ) ;
#5223=PLANE ( 'NONE',  #4409 ) ;
#5240=DIRECTION ( 'NONE',  ( -1.000000000000000000, 0.000000000000000000, 0.000000000000000000 ) ) ;
#5274=ORIENTED_EDGE ( 'NONE', *, *, #4563, .F. ) ;
#5286=DIRECTION ( 'NONE',  ( 0.000000000000000000, 0.8772744497699203059, 0.4799891038147465760 ) ) ;
#5288=CIRCLE ( 'NONE', #6098, 5.999999999999999112 ) ;
#5297=DIRECTION ( 'NONE',  ( 0.000000000000000000, -1.000000000000000000, 0.000000000000000000 ) ) ;
#5302=AXIS2_PLACEMENT_3D ( 'NONE', #10548, #734, #4549 ) ;
#5306=EDGE_CURVE ( 'NONE', #9414, #2515, #5824, .T. ) ;
#5326=DIRECTION ( 'NONE',  ( -1.000000000000000000, 0.000000000000000000, -0.000000000000000000 ) ) ;
#5342=VERTEX_POINT ( 'NONE', #73 ) ;
#5346=DIRECTION ( 'NONE',  ( 0.000000000000000000, 0.7900737791495477946, 0.6130117645692876316 ) ) ;
#5362=DIRECTION ( 'NONE',  ( 1.000000000000000000, 3.903127820947815962E-18, 0.000000000000000000 ) ) ;
#5380=ORIENTED_EDGE ( 'NONE', *, *, #4713, .F. ) ;
#5391=EDGE_CURVE ( 'NONE', #10175, #3842, #2127, .T. ) ;
#5420=ORIENTED_EDGE ( 'NONE', *, *, #6145, .T. ) ;
#5435=AXIS2_PLACEMENT_3D ( 'NONE', #8144, #8906, #11925 ) ;
#5445=CARTESIAN_POINT ( 'NONE',  ( -38.00000000000000000, 7.347880794884118750E-16, 5.999999999999999112 ) ) ;
#5462=CARTESIAN_POINT ( 'NONE',  ( 36.00000000000000711, 0.000000000000000000, 5.000000000000000000 ) ) ;
#5513=DIRECTION ( 'NONE',  ( -1.000000000000000000, -3.903127820947815962E-18, 0.000000000000000000 ) ) ;
#5520=ORIENTED_EDGE ( 'NONE', *, *, #502, .F. ) ;
#5557=AXIS2_PLACEMENT_3D ( 'NONE', #1774, #6671, #5851 ) ;
#5563=CARTESIAN_POINT ( 'NONE',  ( 45.00000000000000000, -3.185523555419108810, 3.853886308373663638 ) ) ;
#5572=ORIENTED_EDGE ( 'NONE', *, *, #5768, .T. ) ;
#5605=VECTOR ( 'NONE', #1984, 1000.000000000000000 ) ;
#5612=ADVANCED_FACE ( 'NONE', ( #10001 ), #1549, .F. ) ;
#5621=( GEOMETRIC_REPRESENTATION_CONTEXT ( 3 ) GLOBAL_UNCERTAINTY_ASSIGNED_CONTEXT ( ( #2521 ) ) GLOBAL_UNIT_ASSIGNED_CONTEXT ( ( #1562, #4446, #12244 ) ) REPRESENTATION_CONTEXT ( 'NONE', 'WORKASPACE' ) );
#5622=CIRCLE ( 'NONE', #11214, 5.000000000000000000 ) ;
#5626=CARTESIAN_POINT ( 'NONE',  ( 45.00000000000000000, 6.123233995736765296E-16, -5.000000000000000000 ) ) ;
#5648=VECTOR ( 'NONE', #3668, 1000.000000000000000 ) ;
#5650=FACE_OUTER_BOUND ( 'NONE', #11569, .T. ) ;
#5685=ORIENTED_EDGE ( 'NONE', *, *, #785, .T. ) ;
#5717=DIRECTION ( 'NONE',  ( -0.000000000000000000, 0.000000000000000000, 1.000000000000000000 ) ) ;
#5729=ORIENTED_EDGE ( 'NONE', *, *, #1629, .F. ) ;
#5737=ORIENTED_EDGE ( 'NONE', *, *, #3796, .T. ) ;
#5764=ORIENTED_EDGE ( 'NONE', *, *, #8557, .F. ) ;
#5768=EDGE_CURVE ( 'NONE', #2515, #9277, #1936, .T. ) ;
#5770=EDGE_CURVE ( 'NONE', #317, #11797, #10690, .T. ) ;
#5777=STYLED_ITEM('',(#12412),#259);
#5791=VECTOR ( 'NONE', #3263, 1000.000000000000000 ) ;
#5824=LINE ( 'NONE', #5563, #8294 ) ;
#5847=PRODUCT_DEFINITION_FORMATION_WITH_SPECIFIED_SOURCE ( 'ANY', '', #9932, .NOT_KNOWN. ) ;
#5851=DIRECTION ( 'NONE',  ( 0.000000000000000000, 0.8772744497699203059, 0.4799891038147465760 ) ) ;
#5865=ADVANCED_FACE ( 'NONE', ( #3068, #9692 ), #10684, .F. ) ;
#5871=ADVANCED_FACE ( 'NONE', ( #3987 ), #8690, .T. ) ;
#5891=FACE_OUTER_BOUND ( 'NONE', #10325, .T. ) ;
#5902=CARTESIAN_POINT ( 'NONE',  ( 43.00000000000000000, -3.792354139917828881, -2.942456469932581253 ) ) ;
#5915=CARTESIAN_POINT ( 'NONE',  ( 29.56763832957518545, 0.000000000000000000, 1.500000000000000000 ) ) ;
#5930=EDGE_CURVE ( 'NONE', #3666, #733, #9418, .T. ) ;
#5937=EDGE_CURVE ( 'NONE', #8121, #4854, #2413, .T. ) ;
#5943=LINE ( 'NONE', #3188, #7073 ) ;
#5950=CARTESIAN_POINT ( 'NONE',  ( 45.00000000000000000, 4.769696007084727185, -1.500000000000000000 ) ) ;
#5952=DIRECTION ( 'NONE',  ( -1.000000000000000000, -0.000000000000000000, -0.000000000000000000 ) ) ;
#5956=EDGE_CURVE ( 'NONE', #504, #4854, #6634, .T. ) ;
#5958=ADVANCED_FACE ( 'NONE', ( #2348 ), #3307, .T. ) ;
#5967=VECTOR ( 'NONE', #6181, 1000.000000000000114 ) ;
#5973=ORIENTED_EDGE ( 'NONE', *, *, #10732, .T. ) ;
#5979=CARTESIAN_POINT ( 'NONE',  ( 37.00000000000000711, -2.432816653220593039, 4.137801726981678030 ) ) ;
#6042=ORIENTED_EDGE ( 'NONE', *, *, #4117, .F. ) ;
#6056=AXIS2_PLACEMENT_3D ( 'NONE', #212, #4035, #8864 ) ;
#6059=VERTEX_POINT ( 'NONE', #2295 ) ;
#6063=CIRCLE ( 'NONE', #669, 5.999999999999999112 ) ;
#6079=AXIS2_PLACEMENT_3D ( 'NONE', #5094, #10850, #11706 ) ;
#6087=DIRECTION ( 'NONE',  ( -1.000000000000000000, -3.903127820947815962E-18, 0.000000000000000000 ) ) ;
#6098=AXIS2_PLACEMENT_3D ( 'NONE', #7207, #6203, #8205 ) ;
#6100=AXIS2_PLACEMENT_3D ( 'NONE', #4383, #8212, #12008 ) ;
#6113=VERTEX_POINT ( 'NONE', #1727 ) ;
#6119=CARTESIAN_POINT ( 'NONE',  ( 43.00000000000000000, 0.000000000000000000, 5.000000000000000000 ) ) ;
#6131=DIRECTION ( 'NONE',  ( 0.000000000000000000, 1.000000000000000000, 0.000000000000000000 ) ) ;
#6145=EDGE_CURVE ( 'NONE', #10175, #4256, #9423, .T. ) ;
#6153=CARTESIAN_POINT ( 'NONE',  ( 43.00000000000000000, 6.123233995736765296E-16, -5.000000000000000000 ) ) ;
#6159=VECTOR ( 'NONE', #8395, 1000.000000000000000 ) ;
#6161=CARTESIAN_POINT ( 'NONE',  ( 43.00000000000000000, -3.185523555419110586, 3.853886308373666747 ) ) ;
#6165=CARTESIAN_POINT ( 'NONE',  ( 36.00000000000000711, -4.104405154062230115E-16, -2.224720805914714718E-17 ) ) ;
#6181=DIRECTION ( 'NONE',  ( -2.731402571913187487E-17, -0.5883347247165658933, 0.8086174940555531654 ) ) ;
#6202=ORIENTED_EDGE ( 'NONE', *, *, #11477, .F. ) ;
#6203=DIRECTION ( 'NONE',  ( -1.000000000000000000, 0.000000000000000000, 0.000000000000000000 ) ) ;
#6217=ORIENTED_EDGE ( 'NONE', *, *, #7379, .T. ) ;
#6222=AXIS2_PLACEMENT_3D ( 'NONE', #5057, #4162, #7991 ) ;
#6224=EDGE_CURVE ( 'NONE', #1927, #7407, #3628, .T. ) ;
#6227=AXIS2_PLACEMENT_3D ( 'NONE', #12115, #8275, #6569 ) ;
#6234=ORIENTED_EDGE ( 'NONE', *, *, #502, .T. ) ;
#6241=AXIS2_PLACEMENT_3D ( 'NONE', #6165, #8987, #4158 ) ;
#6244=DIRECTION ( 'NONE',  ( 0.000000000000000000, 0.000000000000000000, 1.000000000000000000 ) ) ;
#6281=LINE ( 'NONE', #2456, #6159 ) ;
#6284=ORIENTED_EDGE ( 'NONE', *, *, #8797, .F. ) ;
#6327=DIRECTION ( 'NONE',  ( 1.000000000000000000, 3.903127820947815962E-18, 0.000000000000000000 ) ) ;
#6345=DIRECTION ( 'NONE',  ( 1.000000000000000000, 0.000000000000000000, 0.000000000000000000 ) ) ;
#6366=ORIENTED_EDGE ( 'NONE', *, *, #3796, .F. ) ;
#6371=DIRECTION ( 'NONE',  ( 0.000000000000000000, 0.000000000000000000, 1.000000000000000000 ) ) ;
#6405=AXIS2_PLACEMENT_3D ( 'NONE', #955, #207, #10712 ) ;
#6409=PLANE ( 'NONE',  #9380 ) ;
#6417=LINE ( 'NONE', #846, #3458 ) ;
#6437=ORIENTED_EDGE ( 'NONE', *, *, #5956, .F. ) ;
#6448=DIRECTION ( 'NONE',  ( 0.000000000000000000, 0.8772744497699203059, 0.4799891038147465760 ) ) ;
#6450=VERTEX_POINT ( 'NONE', #2453 ) ;
#6477=CIRCLE ( 'NONE', #8080, 4.799999999999998934 ) ;
#6499=ADVANCED_FACE ( 'NONE', ( #748 ), #12182, .T. ) ;
#6509=ORIENTED_EDGE ( 'NONE', *, *, #11100, .F. ) ;
#6515=DIRECTION ( 'NONE',  ( 0.000000000000000000, 0.000000000000000000, 1.000000000000000000 ) ) ;
#6542=CARTESIAN_POINT ( 'NONE',  ( -36.00000000000000000, 0.000000000000000000, 0.000000000000000000 ) ) ;
#6563=DIRECTION ( 'NONE',  ( -1.000000000000000000, 0.000000000000000000, 0.000000000000000000 ) ) ;
#6565=ORIENTED_EDGE ( 'NONE', *, *, #1804, .F. ) ;
#6569=DIRECTION ( 'NONE',  ( 0.000000000000000000, 0.8772744497699203059, 0.4799891038147465760 ) ) ;
#6598=ORIENTED_EDGE ( 'NONE', *, *, #10283, .T. ) ;
#6607=VECTOR ( 'NONE', #1999, 1000.000000000000000 ) ;
#6634=CIRCLE ( 'NONE', #7827, 5.000000000000000000 ) ;
#6654=AXIS2_PLACEMENT_3D ( 'NONE', #3523, #8282, #7342 ) ;
#6662=FACE_OUTER_BOUND ( 'NONE', #2899, .T. ) ;
#6663=EDGE_CURVE ( 'NONE', #3666, #344, #8760, .T. ) ;
#6671=DIRECTION ( 'NONE',  ( -1.000000000000000000, 0.000000000000000000, 0.000000000000000000 ) ) ;
#6674=ORIENTED_EDGE ( 'NONE', *, *, #10283, .F. ) ;
#6692=ORIENTED_EDGE ( 'NONE', *, *, #285, .F. ) ;
#6695=ORIENTED_EDGE ( 'NONE', *, *, #3117, .T. ) ;
#6708=CARTESIAN_POINT ( 'NONE',  ( 42.00000000000000000, -3.792354139917828881, -2.942456469932581253 ) ) ;
#6724=ORIENTED_EDGE ( 'NONE', *, *, #12236, .F. ) ;
#6736=ORIENTED_EDGE ( 'NONE', *, *, #5770, .T. ) ;
#6757=CARTESIAN_POINT ( 'NONE',  ( -36.00000000000000000, 0.000000000000000000, 0.000000000000000000 ) ) ;
#6817=AXIS2_PLACEMENT_3D ( 'NONE', #1848, #3031, #8785 ) ;
#6822=CARTESIAN_POINT ( 'NONE',  ( 42.00000000000000000, -2.824006678639516377, 3.881363971466655904 ) ) ;
#6827=CARTESIAN_POINT ( 'NONE',  ( 45.00000000000000000, 0.000000000000000000, 0.000000000000000000 ) ) ;
#6857=LINE ( 'NONE', #3218, #762 ) ;
#6866=EDGE_LOOP ( 'NONE', ( #5380, #6217, #512, #6202 ) ) ;
#6916=ORIENTED_EDGE ( 'NONE', *, *, #12265, .F. ) ;
#6954=ORIENTED_EDGE ( 'NONE', *, *, #5930, .T. ) ;
#6956=CARTESIAN_POINT ( 'NONE',  ( 43.00000000000000000, 3.792354139917828437, 2.942456469932579921 ) ) ;
#6977=CARTESIAN_POINT ( 'NONE',  ( 36.00000000000000711, -2.534184013771451305, 4.310210132272582761 ) ) ;
#7008=AXIS2_PLACEMENT_3D ( 'NONE', #11117, #11246, #6371 ) ;
#7033=DIRECTION ( 'NONE',  ( -1.000000000000000000, -0.000000000000000000, -0.000000000000000000 ) ) ;
#7073=VECTOR ( 'NONE', #4176, 1000.000000000000000 ) ;
#7083=FACE_OUTER_BOUND ( 'NONE', #8816, .T. ) ;
#7123=DIRECTION ( 'NONE',  ( -0.000000000000000000, -0.8916709834801178625, -0.4526840589413320126 ) ) ;
#7150=LINE ( 'NONE', #1211, #7836 ) ;
#7177=DIRECTION ( 'NONE',  ( 1.000000000000000000, 0.000000000000000000, 0.000000000000000000 ) ) ;
#7193=AXIS2_PLACEMENT_3D ( 'NONE', #12081, #3532, #5346 ) ;
#7207=CARTESIAN_POINT ( 'NONE',  ( -38.00000000000000000, 0.000000000000000000, 0.000000000000000000 ) ) ;
#7234=CIRCLE ( 'NONE', #11608, 4.799999999999998934 ) ;
#7281=DIRECTION ( 'NONE',  ( 0.000000000000000000, -1.000000000000000000, 0.000000000000000000 ) ) ;
#7282=ORIENTED_EDGE ( 'NONE', *, *, #11525, .F. ) ;
#7288=CARTESIAN_POINT ( 'NONE',  ( 42.00000000000000000, 3.792354139917828437, 2.942456469932579921 ) ) ;
#7310=DIRECTION ( 'NONE',  ( 1.000000000000000000, -0.000000000000000000, -0.000000000000000000 ) ) ;
#7342=DIRECTION ( 'NONE',  ( 0.000000000000000000, 0.000000000000000000, 1.000000000000000000 ) ) ;
#7348=ORIENTED_EDGE ( 'NONE', *, *, #3674, .T. ) ;
#7354=EDGE_LOOP ( 'NONE', ( #4993, #12281, #2423, #2929 ) ) ;
#7372=CIRCLE ( 'NONE', #5167, 5.000000000000000000 ) ;
#7373=DIRECTION ( 'NONE',  ( 0.000000000000000000, 0.8772744497699204169, 0.4799891038147465205 ) ) ;
#7379=EDGE_CURVE ( 'NONE', #10072, #4240, #2349, .T. ) ;
#7381=EDGE_CURVE ( 'NONE', #4485, #504, #1172, .T. ) ;
#7382=DIRECTION ( 'NONE',  ( -1.000000000000000000, -0.000000000000000000, -0.000000000000000000 ) ) ;
#7392=VERTEX_POINT ( 'NONE', #12223 ) ;
#7406=EDGE_LOOP ( 'NONE', ( #3223, #12248, #3955, #1381 ) ) ;
#7407=VERTEX_POINT ( 'NONE', #9360 ) ;
#7416=CIRCLE ( 'NONE', #10602, 5.000000000000000000 ) ;
#7418=ORIENTED_EDGE ( 'NONE', *, *, #12104, .F. ) ;
#7419=VERTEX_POINT ( 'NONE', #7546 ) ;
#7452=EDGE_LOOP ( 'NONE', ( #5685, #9807, #9365, #2112, #4737, #1864, #1507, #9247, #6736, #1627, #8505, #10488 ) ) ;
#7478=EDGE_CURVE ( 'NONE', #5131, #7419, #10478, .T. ) ;
#7491=EDGE_LOOP ( 'NONE', ( #8033, #12018 ) ) ;
#7519=EDGE_CURVE ( 'NONE', #4854, #5131, #10037, .T. ) ;
#7525=CARTESIAN_POINT ( 'NONE',  ( 45.00000000000000000, 0.000000000000000000, 0.000000000000000000 ) ) ;
#7546=CARTESIAN_POINT ( 'NONE',  ( 36.00000000000000711, -2.432816653220593039, 4.137801726981678030 ) ) ;
#7548=ORIENTED_EDGE ( 'NONE', *, *, #9680, .F. ) ;
#7555=VERTEX_POINT ( 'NONE', #3525 ) ;
#7571=DIRECTION ( 'NONE',  ( 0.000000000000000000, 0.7900737791495477946, 0.6130117645692876316 ) ) ;
#7576=VECTOR ( 'NONE', #3342, 999.9999999999998863 ) ;
#7581=DIRECTION ( 'NONE',  ( -2.731402571913187487E-17, -0.5883347247165658933, 0.8086174940555532764 ) ) ;
#7602=ORIENTED_EDGE ( 'NONE', *, *, #11881, .T. ) ;
#7619=VECTOR ( 'NONE', #12225, 1000.000000000000000 ) ;
#7623=DIRECTION ( 'NONE',  ( 1.000000000000000000, -0.000000000000000000, -0.000000000000000000 ) ) ;
#7641=LINE ( 'NONE', #5626, #9450 ) ;
#7690=ORIENTED_EDGE ( 'NONE', *, *, #4713, .T. ) ;
#7695=CARTESIAN_POINT ( 'NONE',  ( 43.00000000000000000, -3.058102613202345665, 3.699730856038719207 ) ) ;
#7700=ADVANCED_FACE ( 'NONE', ( #5650 ), #2704, .T. ) ;
#7731=ORIENTED_EDGE ( 'NONE', *, *, #662, .T. ) ;
#7750=EDGE_CURVE ( 'NONE', #2996, #1270, #7985, .T. ) ;
#7751=DIRECTION ( 'NONE',  ( -1.000000000000000000, -0.000000000000000000, -0.000000000000000000 ) ) ;
#7758=DIRECTION ( 'NONE',  ( 0.000000000000000000, 0.7900737791495477946, 0.6130117645692876316 ) ) ;
#7769=DIRECTION ( 'NONE',  ( -1.472782982004545120E-17, -0.8086174940555532764, -0.5883347247165658933 ) ) ;
#7778=AXIS2_PLACEMENT_3D ( 'NONE', #2069, #6563, #1122 ) ;
#7784=VECTOR ( 'NONE', #1610, 1000.000000000000000 ) ;
#7824=VECTOR ( 'NONE', #1868, 1000.000000000000000 ) ;
#7827=AXIS2_PLACEMENT_3D ( 'NONE', #4481, #10915, #8248 ) ;
#7836=VECTOR ( 'NONE', #11887, 1000.000000000000000 ) ;
#7840=CARTESIAN_POINT ( 'NONE',  ( -38.00000000000000000, 0.000000000000000000, -5.999999999999999112 ) ) ;
#7855=CIRCLE ( 'NONE', #8445, 5.000000000000000000 ) ;
#7884=AXIS2_PLACEMENT_3D ( 'NONE', #7972, #10041, #5286 ) ;
#7885=LINE ( 'NONE', #2064, #6607 ) ;
#7933=ORIENTED_EDGE ( 'NONE', *, *, #2944, .F. ) ;
#7937=PRODUCT_DEFINITION ( 'UNKNOWN', '', #5847, #9029 ) ;
#7938=APPLICATION_CONTEXT ( 'automotive_design' ) ;
#7943=DIRECTION ( 'NONE',  ( -1.000000000000000000, -0.000000000000000000, -0.000000000000000000 ) ) ;
#7972=CARTESIAN_POINT ( 'NONE',  ( 36.00000000000000711, -4.104405154062230115E-16, -2.224720805914714718E-17 ) ) ;
#7985=CIRCLE ( 'NONE', #9184, 5.000000000000000000 ) ;
#7991=DIRECTION ( 'NONE',  ( 0.000000000000000000, -1.000000000000000000, 0.000000000000000000 ) ) ;
#7998=ORIENTED_EDGE ( 'NONE', *, *, #8074, .F. ) ;
#8028=FACE_OUTER_BOUND ( 'NONE', #8325, .T. ) ;
#8033=ORIENTED_EDGE ( 'NONE', *, *, #3117, .F. ) ;
#8064=VECTOR ( 'NONE', #9893, 1000.000000000000000 ) ;
#8074=EDGE_CURVE ( 'NONE', #11797, #11945, #3053, .T. ) ;
#8080=AXIS2_PLACEMENT_3D ( 'NONE', #9111, #4392, #12078 ) ;
#8090=CARTESIAN_POINT ( 'NONE',  ( 43.00000000000000000, -2.824006678639516377, 3.881363971466655904 ) ) ;
#8105=CARTESIAN_POINT ( 'NONE',  ( 36.00000000000000711, -2.432816653220593039, 4.137801726981678030 ) ) ;
#8121=VERTEX_POINT ( 'NONE', #6977 ) ;
#8144=CARTESIAN_POINT ( 'NONE',  ( 37.00000000000000711, -4.104405154062230115E-16, -2.224720805914714718E-17 ) ) ;
#8158=CARTESIAN_POINT ( 'NONE',  ( 45.00000000000000000, 0.000000000000000000, 5.000000000000000000 ) ) ;
#8162=ORIENTED_EDGE ( 'NONE', *, *, #6663, .F. ) ;
#8186=EDGE_LOOP ( 'NONE', ( #10861, #1247, #2639, #7998 ) ) ;
#8198=ORIENTED_EDGE ( 'NONE', *, *, #11525, .T. ) ;
#8205=DIRECTION ( 'NONE',  ( 0.000000000000000000, 0.000000000000000000, 1.000000000000000000 ) ) ;
#8212=DIRECTION ( 'NONE',  ( -1.000000000000000000, 9.497745524640252240E-18, 1.039762770660628461E-17 ) ) ;
#8219=LINE ( 'NONE', #8158, #9822 ) ;
#8230=VECTOR ( 'NONE', #11763, 999.9999999999998863 ) ;
#8235=AXIS2_PLACEMENT_3D ( 'NONE', #6542, #9724, #4954 ) ;
#8248=DIRECTION ( 'NONE',  ( 0.000000000000000000, 0.000000000000000000, 1.000000000000000000 ) ) ;
#8256=AXIS2_PLACEMENT_3D ( 'NONE', #10014, #5952, #8838 ) ;
#8266=LINE ( 'NONE', #5445, #1199 ) ;
#8273=DIRECTION ( 'NONE',  ( 1.000000000000000000, 3.903127820947815962E-18, 0.000000000000000000 ) ) ;
#8275=DIRECTION ( 'NONE',  ( 1.000000000000000000, -0.000000000000000000, 0.000000000000000000 ) ) ;
#8282=DIRECTION ( 'NONE',  ( 1.000000000000000000, -0.000000000000000000, -0.000000000000000000 ) ) ;
#8293=FACE_OUTER_BOUND ( 'NONE', #503, .T. ) ;
#8294=VECTOR ( 'NONE', #11311, 1000.000000000000000 ) ;
#8325=EDGE_LOOP ( 'NONE', ( #4531, #7418, #10236, #856, #11562, #9720, #4293, #973, #6692, #6674, #320, #11029 ) ) ;
#8330=ADVANCED_FACE ( 'NONE', ( #4526 ), #4662, .T. ) ;
#8342=( NAMED_UNIT ( * ) PLANE_ANGLE_UNIT ( ) SI_UNIT ( $, .RADIAN. ) );
#8349=CARTESIAN_POINT ( 'NONE',  ( 36.00000000000000711, -2.172883482918394282, 4.280020720704565740 ) ) ;
#8350=EDGE_LOOP ( 'NONE', ( #2201, #4578, #11366, #6509 ) ) ;
#8354=VERTEX_POINT ( 'NONE', #9295 ) ;
#8356=DIRECTION ( 'NONE',  ( -1.000000000000000000, 0.000000000000000000, 0.000000000000000000 ) ) ;
#8380=ORIENTED_EDGE ( 'NONE', *, *, #5183, .T. ) ;
#8392=CIRCLE ( 'NONE', #11374, 5.000000000000000000 ) ;
#8395=DIRECTION ( 'NONE',  ( 1.000000000000000000, 0.000000000000000000, 0.000000000000000000 ) ) ;
#8409=AXIS2_PLACEMENT_3D ( 'NONE', #11080, #10260, #11132 ) ;
#8431=CIRCLE ( 'NONE', #6227, 4.799999999999999822 ) ;
#8445=AXIS2_PLACEMENT_3D ( 'NONE', #3303, #9981, #5297 ) ;
#8462=ADVANCED_FACE ( 'NONE', ( #11575 ), #1025, .T. ) ;
#8490=EDGE_CURVE ( 'NONE', #1270, #2996, #8600, .T. ) ;
#8494=ORIENTED_EDGE ( 'NONE', *, *, #4270, .F. ) ;
#8505=ORIENTED_EDGE ( 'NONE', *, *, #11233, .T. ) ;
#8557=EDGE_CURVE ( 'NONE', #6059, #11661, #10184, .T. ) ;
#8568=DIRECTION ( 'NONE',  ( -1.000000000000000000, -3.903127820947815962E-18, 0.000000000000000000 ) ) ;
#8600=CIRCLE ( 'NONE', #6405, 5.000000000000000000 ) ;
#8610=CARTESIAN_POINT ( 'NONE',  ( 37.00000000000000711, -2.172883482918394282, 4.280020720704565740 ) ) ;
#8620=CARTESIAN_POINT ( 'NONE',  ( -38.00000000000000000, 0.000000000000000000, -5.999999999999999112 ) ) ;
#8623=( GEOMETRIC_REPRESENTATION_CONTEXT ( 3 ) GLOBAL_UNCERTAINTY_ASSIGNED_CONTEXT ( ( #3658 ) ) GLOBAL_UNIT_ASSIGNED_CONTEXT ( ( #4312, #1452, #1510 ) ) REPRESENTATION_CONTEXT ( 'NONE', 'WORKASPACE' ) );
#8690=CYLINDRICAL_SURFACE ( 'NONE', #1422, 4.799999999999998934 ) ;
#8700=CARTESIAN_POINT ( 'NONE',  ( 43.00000000000000000, -2.824006678639516377, 3.881363971466655904 ) ) ;
#8703=CARTESIAN_POINT ( 'NONE',  ( 43.00000000000000000, 3.903127820947864496E-18, 0.000000000000000000 ) ) ;
#8705=ORIENTED_EDGE ( 'NONE', *, *, #1116, .T. ) ;
#8721=CYLINDRICAL_SURFACE ( 'NONE', #5557, 4.799999999999999822 ) ;
#8738=EDGE_CURVE ( 'NONE', #9966, #1854, #11788, .T. ) ;
#8760=LINE ( 'NONE', #5123, #5791 ) ;
#8785=DIRECTION ( 'NONE',  ( 0.000000000000000000, 0.000000000000000000, -1.000000000000000000 ) ) ;
#8797=EDGE_CURVE ( 'NONE', #4256, #4485, #8951, .T. ) ;
#8816=EDGE_LOOP ( 'NONE', ( #2925, #7731, #3147, #6565 ) ) ;
#8830=EDGE_CURVE ( 'NONE', #8354, #2097, #7416, .T. ) ;
#8838=DIRECTION ( 'NONE',  ( 0.000000000000000000, 0.000000000000000000, 1.000000000000000000 ) ) ;
#8864=DIRECTION ( 'NONE',  ( 1.000000000000000000, 0.000000000000000000, 0.000000000000000000 ) ) ;
#8885=DIRECTION ( 'NONE',  ( 0.000000000000000000, 0.000000000000000000, 1.000000000000000000 ) ) ;
#8887=CIRCLE ( 'NONE', #6079, 5.000000000000000000 ) ;
#8898=CIRCLE ( 'NONE', #3906, 5.000000000000000000 ) ;
#8906=DIRECTION ( 'NONE',  ( -1.000000000000000000, 0.000000000000000000, 0.000000000000000000 ) ) ;
#8922=ORIENTED_EDGE ( 'NONE', *, *, #3699, .F. ) ;
#8933=ORIENTED_EDGE ( 'NONE', *, *, #4270, .T. ) ;
#8939=EDGE_CURVE ( 'NONE', #9414, #7555, #920, .T. ) ;
#8951=LINE ( 'NONE', #5950, #10795 ) ;
#8955=ORIENTED_EDGE ( 'NONE', *, *, #595, .T. ) ;
#8983=DIRECTION ( 'NONE',  ( 0.000000000000000000, 0.5068368027542899945, -0.8620420264545162192 ) ) ;
#8987=DIRECTION ( 'NONE',  ( 1.000000000000000000, -0.000000000000000000, 0.000000000000000000 ) ) ;
#8997=ADVANCED_FACE ( 'NONE', ( #2438 ), #12344, .F. ) ;
#9029=PRODUCT_DEFINITION_CONTEXT ( 'detailed design', #493, 'design' ) ;
#9034=MECHANICAL_DESIGN_GEOMETRIC_PRESENTATION_REPRESENTATION('',(#4028),#5621);
#9048=DIRECTION ( 'NONE',  ( -1.000000000000000000, -0.000000000000000000, -0.000000000000000000 ) ) ;
#9058=PLANE ( 'NONE',  #5220 ) ;
#9061=ORIENTED_EDGE ( 'NONE', *, *, #1536, .F. ) ;
#9071=ORIENTED_EDGE ( 'NONE', *, *, #914, .T. ) ;
#9092=CARTESIAN_POINT ( 'NONE',  ( 42.00000000000000000, 4.814824860968089633E-32, 0.000000000000000000 ) ) ;
#9111=CARTESIAN_POINT ( 'NONE',  ( 43.00000000000000000, 3.903127820947864496E-18, 0.000000000000000000 ) ) ;
#9143=DIRECTION ( 'NONE',  ( 0.000000000000000000, 0.7900737791495477946, 0.6130117645692876316 ) ) ;
#9178=CARTESIAN_POINT ( 'NONE',  ( 45.00000000000000000, -2.534184013771451305, 4.310210132272580097 ) ) ;
#9184=AXIS2_PLACEMENT_3D ( 'NONE', #12314, #3762, #11319 ) ;
#9191=ORIENTED_EDGE ( 'NONE', *, *, #484, .T. ) ;
#9203=SURFACE_SIDE_STYLE ('',( #693 ) ) ;
#9205=DIRECTION ( 'NONE',  ( 0.000000000000000000, 0.7900737791495477946, 0.6130117645692876316 ) ) ;
#9210=ORIENTED_EDGE ( 'NONE', *, *, #10825, .F. ) ;
#9247=ORIENTED_EDGE ( 'NONE', *, *, #1536, .T. ) ;
#9268=CARTESIAN_POINT ( 'NONE',  ( 37.00000000000000711, -4.104405154062230115E-16, -2.224720805914714718E-17 ) ) ;
#9277=VERTEX_POINT ( 'NONE', #9977 ) ;
#9282=ADVANCED_FACE ( 'NONE', ( #3348 ), #9058, .F. ) ;
#9295=CARTESIAN_POINT ( 'NONE',  ( -36.00000000000000000, 6.123233995736765296E-16, -5.000000000000000000 ) ) ;
#9315=EDGE_CURVE ( 'NONE', #1890, #1765, #5622, .T. ) ;
#9349=CARTESIAN_POINT ( 'NONE',  ( 42.00000000000000000, 4.769696007084728073, 1.500000000000000444 ) ) ;
#9360=CARTESIAN_POINT ( 'NONE',  ( -36.00000000000000000, 0.000000000000000000, -5.999999999999999112 ) ) ;
#9365=ORIENTED_EDGE ( 'NONE', *, *, #914, .F. ) ;
#9380=AXIS2_PLACEMENT_3D ( 'NONE', #1661, #2523, #6345 ) ;
#9381=DIRECTION ( 'NONE',  ( -1.000000000000000000, -3.903127820947815962E-18, 0.000000000000000000 ) ) ;
#9404=EDGE_LOOP ( 'NONE', ( #2850, #9191, #9992, #10693 ) ) ;
#9414=VERTEX_POINT ( 'NONE', #1664 ) ;
#9415=EDGE_LOOP ( 'NONE', ( #1628, #12122, #10388, #6366 ) ) ;
#9418=CIRCLE ( 'NONE', #6222, 5.000000000000000000 ) ;
#9419=ORIENTED_EDGE ( 'NONE', *, *, #5768, .F. ) ;
#9423=LINE ( 'NONE', #4018, #5216 ) ;
#9428=VERTEX_POINT ( 'NONE', #9349 ) ;
#9431=CARTESIAN_POINT ( 'NONE',  ( 37.00000000000000711, 6.799999999999998046, -1.500000000000000000 ) ) ;
#9432=DIRECTION ( 'NONE',  ( 2.817067928751547788E-17, 0.6371047110838219396, -0.7707772616747329275 ) ) ;
#9450=VECTOR ( 'NONE', #4746, 1000.000000000000000 ) ;
#9452=PLANE ( 'NONE',  #7778 ) ;
#9458=ADVANCED_BREP_SHAPE_REPRESENTATION ( '', ( #259, #6056 ), #8623 ) ;
#9481=DIRECTION ( 'NONE',  ( 0.000000000000000000, 0.8772744497699203059, 0.4799891038147465760 ) ) ;
#9509=DIRECTION ( 'NONE',  ( 0.000000000000000000, -1.000000000000000000, 0.000000000000000000 ) ) ;
#9536=DIRECTION ( 'NONE',  ( 1.000000000000000000, 0.000000000000000000, 0.000000000000000000 ) ) ;
#9609=EDGE_LOOP ( 'NONE', ( #12091, #8494, #9419, #9735 ) ) ;
#9625=COLOUR_RGB ( '',0.8941176470588234615, 0.8941176470588234615, 0.8941176470588234615 ) ;
#9628=VECTOR ( 'NONE', #11876, 1000.000000000000114 ) ;
#9662=CARTESIAN_POINT ( 'NONE',  ( 37.00000000000000711, -2.534184013771451305, 4.310210132272582761 ) ) ;
#9680=EDGE_CURVE ( 'NONE', #8121, #7419, #3962, .T. ) ;
#9692=FACE_OUTER_BOUND ( 'NONE', #10210, .T. ) ;
#9715=FACE_OUTER_BOUND ( 'NONE', #8350, .T. ) ;
#9720=ORIENTED_EDGE ( 'NONE', *, *, #3959, .F. ) ;
#9724=DIRECTION ( 'NONE',  ( -1.000000000000000000, 0.000000000000000000, 0.000000000000000000 ) ) ;
#9735=ORIENTED_EDGE ( 'NONE', *, *, #5306, .F. ) ;
#9807=ORIENTED_EDGE ( 'NONE', *, *, #10981, .T. ) ;
#9822=VECTOR ( 'NONE', #9048, 1000.000000000000000 ) ;
#9893=DIRECTION ( 'NONE',  ( 0.000000000000000000, -1.000000000000000000, 0.000000000000000000 ) ) ;
#9913=LINE ( 'NONE', #11026, #11753 ) ;
#9932=PRODUCT ( 'hub', 'hub', '', ( #3970 ) ) ;
#9934=CARTESIAN_POINT ( 'NONE',  ( 37.00000000000000711, -2.172883482918394282, 4.280020720704565740 ) ) ;
#9939=CARTESIAN_POINT ( 'NONE',  ( 36.00000000000000711, -2.172883482918394282, 4.280020720704565740 ) ) ;
#9953=DIRECTION ( 'NONE',  ( -1.000000000000000000, 0.000000000000000000, 0.000000000000000000 ) ) ;
#9966=VERTEX_POINT ( 'NONE', #7840 ) ;
#9977=CARTESIAN_POINT ( 'NONE',  ( 43.00000000000000000, -3.058102613202345665, 3.699730856038719207 ) ) ;
#9981=DIRECTION ( 'NONE',  ( -1.000000000000000000, -3.903127820947815962E-18, 0.000000000000000000 ) ) ;
#9990=DIRECTION ( 'NONE',  ( -1.000000000000000000, -3.903127820947815962E-18, 0.000000000000000000 ) ) ;
#9992=ORIENTED_EDGE ( 'NONE', *, *, #6224, .T. ) ;
#9993=DIRECTION ( 'NONE',  ( 0.000000000000000000, -0.4526840589413320126, 0.8916709834801178625 ) ) ;
#10001=FACE_OUTER_BOUND ( 'NONE', #3384, .T. ) ;
#10014=CARTESIAN_POINT ( 'NONE',  ( 45.00000000000000000, 0.000000000000000000, 0.000000000000000000 ) ) ;
#10029=FACE_OUTER_BOUND ( 'NONE', #335, .T. ) ;
#10034=CIRCLE ( 'NONE', #6241, 4.799999999999999822 ) ;
#10037=LINE ( 'NONE', #646, #7576 ) ;
#10041=DIRECTION ( 'NONE',  ( 1.000000000000000000, -0.000000000000000000, 0.000000000000000000 ) ) ;
#10072=VERTEX_POINT ( 'NONE', #5902 ) ;
#10074=ADVANCED_FACE ( 'NONE', ( #9715 ), #4946, .T. ) ;
#10075=CARTESIAN_POINT ( 'NONE',  ( 43.00000000000000000, -3.058102613202345665, 3.699730856038719207 ) ) ;
#10084=DIRECTION ( 'NONE',  ( -0.000000000000000000, 0.000000000000000000, 1.000000000000000000 ) ) ;
#10104=CARTESIAN_POINT ( 'NONE',  ( 45.00000000000000000, 0.000000000000000000, 0.000000000000000000 ) ) ;
#10109=VERTEX_POINT ( 'NONE', #8090 ) ;
#10112=VERTEX_POINT ( 'NONE', #1370 ) ;
#10121=ORIENTED_EDGE ( 'NONE', *, *, #1116, .F. ) ;
#10124=ORIENTED_EDGE ( 'NONE', *, *, #7379, .F. ) ;
#10127=EDGE_CURVE ( 'NONE', #3842, #9428, #11871, .T. ) ;
#10138=CARTESIAN_POINT ( 'NONE',  ( 37.00000000000000711, -2.432816653220593039, 4.137801726981678030 ) ) ;
#10175=VERTEX_POINT ( 'NONE', #3201 ) ;
#10184=CIRCLE ( 'NONE', #8409, 5.000000000000000000 ) ;
#10210=EDGE_LOOP ( 'NONE', ( #6042, #11645 ) ) ;
#10216=ADVANCED_FACE ( 'NONE', ( #7083 ), #5075, .T. ) ;
#10226=LINE ( 'NONE', #8349, #5648 ) ;
#10236=ORIENTED_EDGE ( 'NONE', *, *, #4554, .F. ) ;
#10256=CARTESIAN_POINT ( 'NONE',  ( 43.00000000000000000, 0.000000000000000000, 0.000000000000000000 ) ) ;
#10260=DIRECTION ( 'NONE',  ( -1.000000000000000000, 0.000000000000000000, 0.000000000000000000 ) ) ;
#10277=EDGE_CURVE ( 'NONE', #9428, #11661, #3561, .T. ) ;
#10283=EDGE_CURVE ( 'NONE', #4256, #11604, #7372, .T. ) ;
#10312=CARTESIAN_POINT ( 'NONE',  ( 42.00000000000000000, 6.123233995736765296E-16, -5.000000000000000000 ) ) ;
#10325=EDGE_LOOP ( 'NONE', ( #4740, #11454, #3006, #4635 ) ) ;
#10328=EDGE_CURVE ( 'NONE', #5131, #5049, #12339, .T. ) ;
#10355=LINE ( 'NONE', #8620, #2378 ) ;
#10357=CIRCLE ( 'NONE', #3583, 4.799999999999998934 ) ;
#10388=ORIENTED_EDGE ( 'NONE', *, *, #4166, .T. ) ;
#10391=ORIENTED_EDGE ( 'NONE', *, *, #5937, .T. ) ;
#10411=DIRECTION ( 'NONE',  ( 0.000000000000000000, -1.000000000000000000, 0.000000000000000000 ) ) ;
#10419=LINE ( 'NONE', #1866, #5605 ) ;
#10420=DIRECTION ( 'NONE',  ( 2.817067928751547788E-17, 0.6371047110838219396, -0.7707772616747329275 ) ) ;
#10439=LINE ( 'NONE', #6822, #5967 ) ;
#10461=CYLINDRICAL_SURFACE ( 'NONE', #2035, 5.000000000000000000 ) ;
#10468=ADVANCED_FACE ( 'NONE', ( #2001 ), #9452, .T. ) ;
#10478=LINE ( 'NONE', #4540, #3369 ) ;
#10480=ORIENTED_EDGE ( 'NONE', *, *, #10508, .T. ) ;
#10484=CARTESIAN_POINT ( 'NONE',  ( 42.00000000000000000, -3.058102613202345665, 3.699730856038719207 ) ) ;
#10488=ORIENTED_EDGE ( 'NONE', *, *, #8557, .T. ) ;
#10496=CARTESIAN_POINT ( 'NONE',  ( 45.00000000000000000, -2.263420294706659952, 4.458354917400590089 ) ) ;
#10508=EDGE_CURVE ( 'NONE', #88, #344, #10439, .T. ) ;
#10548=CARTESIAN_POINT ( 'NONE',  ( 37.00000000000000711, -4.104405154062230115E-16, -2.224720805914714718E-17 ) ) ;
#10571=FACE_OUTER_BOUND ( 'NONE', #4211, .T. ) ;
#10573=ORIENTED_EDGE ( 'NONE', *, *, #11723, .T. ) ;
#10602=AXIS2_PLACEMENT_3D ( 'NONE', #260, #11741, #4073 ) ;
#10635=CARTESIAN_POINT ( 'NONE',  ( 42.00000000000000000, 4.769696007084728073, -1.500000000000000444 ) ) ;
#10659=AXIS2_PLACEMENT_3D ( 'NONE', #6827, #7943, #4994 ) ;
#10661=DIRECTION ( 'NONE',  ( -1.000000000000000000, 0.000000000000000000, 0.000000000000000000 ) ) ;
#10671=CARTESIAN_POINT ( 'NONE',  ( 42.00000000000000000, -2.824006678639516377, 3.881363971466655904 ) ) ;
#10684=PLANE ( 'NONE',  #1826 ) ;
#10690=CIRCLE ( 'NONE', #5302, 4.799999999999999822 ) ;
#10693=ORIENTED_EDGE ( 'NONE', *, *, #10890, .F. ) ;
#10709=CARTESIAN_POINT ( 'NONE',  ( 37.00000000000000711, -4.210917358895616580, -2.303947698310783387 ) ) ;
#10712=DIRECTION ( 'NONE',  ( 0.000000000000000000, 0.000000000000000000, -1.000000000000000000 ) ) ;
#10732=EDGE_CURVE ( 'NONE', #2996, #733, #2604, .T. ) ;
#10795=VECTOR ( 'NONE', #193, 1000.000000000000000 ) ;
#10825=EDGE_CURVE ( 'NONE', #9277, #10072, #10357, .T. ) ;
#10836=VECTOR ( 'NONE', #68, 1000.000000000000000 ) ;
#10847=CARTESIAN_POINT ( 'NONE',  ( 45.00000000000000000, 0.000000000000000000, 5.000000000000000000 ) ) ;
#10850=DIRECTION ( 'NONE',  ( -1.000000000000000000, -3.903127820947815962E-18, 0.000000000000000000 ) ) ;
#10861=ORIENTED_EDGE ( 'NONE', *, *, #5770, .F. ) ;
#10882=CARTESIAN_POINT ( 'NONE',  ( 29.56763832957518545, 6.799999999999998046, 0.000000000000000000 ) ) ;
#10889=CARTESIAN_POINT ( 'NONE',  ( 37.00000000000000711, -4.104405154062230115E-16, -2.224720805914714718E-17 ) ) ;
#10890=EDGE_CURVE ( 'NONE', #9966, #7407, #10355, .T. ) ;
#10907=DIRECTION ( 'NONE',  ( 0.000000000000000000, 0.000000000000000000, 1.000000000000000000 ) ) ;
#10915=DIRECTION ( 'NONE',  ( -1.000000000000000000, 0.000000000000000000, 0.000000000000000000 ) ) ;
#10933=ORIENTED_EDGE ( 'NONE', *, *, #2399, .F. ) ;
#10937=FILL_AREA_STYLE ('',( #11997 ) ) ;
#10959=AXIS2_PLACEMENT_3D ( 'NONE', #7525, #2757, #4895 ) ;
#10965=DIRECTION ( 'NONE',  ( -1.000000000000000000, 0.000000000000000000, 0.000000000000000000 ) ) ;
#10980=PLANE ( 'NONE',  #2204 ) ;
#10981=EDGE_CURVE ( 'NONE', #5342, #1003, #9913, .T. ) ;
#10994=CARTESIAN_POINT ( 'NONE',  ( 42.00000000000000000, -2.941673623582830022, 4.043087470277766826 ) ) ;
#11006=CARTESIAN_POINT ( 'NONE',  ( 43.00000000000000000, -2.824006678639516377, 3.881363971466655904 ) ) ;
#11026=CARTESIAN_POINT ( 'NONE',  ( 37.00000000000000711, 6.799999999999998046, 0.000000000000000000 ) ) ;
#11029=ORIENTED_EDGE ( 'NONE', *, *, #5391, .T. ) ;
#11066=AXIS2_PLACEMENT_3D ( 'NONE', #10889, #9953, #1378 ) ;
#11072=SURFACE_STYLE_USAGE ( .BOTH. , #9203 ) ;
#11080=CARTESIAN_POINT ( 'NONE',  ( 37.00000000000000711, 0.000000000000000000, 0.000000000000000000 ) ) ;
#11100=EDGE_CURVE ( 'NONE', #1890, #2097, #8219, .T. ) ;
#11107=EDGE_LOOP ( 'NONE', ( #5420, #1088, #9071, #11206 ) ) ;
#11117=CARTESIAN_POINT ( 'NONE',  ( 36.00000000000000711, 0.000000000000000000, 0.000000000000000000 ) ) ;
#11132=DIRECTION ( 'NONE',  ( 0.000000000000000000, 0.000000000000000000, 1.000000000000000000 ) ) ;
#11146=CIRCLE ( 'NONE', #962, 4.799999999999999822 ) ;
#11168=CARTESIAN_POINT ( 'NONE',  ( 45.00000000000000000, 0.000000000000000000, 5.000000000000000000 ) ) ;
#11178=DIRECTION ( 'NONE',  ( 1.000000000000000000, -0.000000000000000000, 0.000000000000000000 ) ) ;
#11206=ORIENTED_EDGE ( 'NONE', *, *, #1804, .T. ) ;
#11214=AXIS2_PLACEMENT_3D ( 'NONE', #4155, #10965, #10907 ) ;
#11233=EDGE_CURVE ( 'NONE', #3600, #6059, #2823, .T. ) ;
#11235=LINE ( 'NONE', #12153, #7619 ) ;
#11246=DIRECTION ( 'NONE',  ( -1.000000000000000000, 0.000000000000000000, 0.000000000000000000 ) ) ;
#11258=DIRECTION ( 'NONE',  ( -1.000000000000000000, -0.000000000000000000, -0.000000000000000000 ) ) ;
#11268=DIRECTION ( 'NONE',  ( 0.000000000000000000, 0.000000000000000000, 1.000000000000000000 ) ) ;
#11308=CARTESIAN_POINT ( 'NONE',  ( 42.00000000000000000, 4.814824860968089633E-32, 0.000000000000000000 ) ) ;
#11311=DIRECTION ( 'NONE',  ( 1.000000000000000000, 0.000000000000000000, 0.000000000000000000 ) ) ;
#11319=DIRECTION ( 'NONE',  ( 0.000000000000000000, 0.000000000000000000, -1.000000000000000000 ) ) ;
#11330=PLANE ( 'NONE',  #12005 ) ;
#11349=ORIENTED_EDGE ( 'NONE', *, *, #10328, .F. ) ;
#11362=( GEOMETRIC_REPRESENTATION_CONTEXT ( 3 ) GLOBAL_UNCERTAINTY_ASSIGNED_CONTEXT ( ( #1920 ) ) GLOBAL_UNIT_ASSIGNED_CONTEXT ( ( #4525, #8342, #763 ) ) REPRESENTATION_CONTEXT ( 'NONE', 'WORKASPACE' ) );
#11366=ORIENTED_EDGE ( 'NONE', *, *, #8830, .T. ) ;
#11368=SHAPE_REPRESENTATION_RELATIONSHIP ( 'NONE' , 'NONE' ,  #678, #9458 ) ;
#11374=AXIS2_PLACEMENT_3D ( 'NONE', #835, #11458, #2906 ) ;
#11425=AXIS2_PLACEMENT_3D ( 'NONE', #8703, #3942, #7758 ) ;
#11433=ADVANCED_FACE ( 'NONE', ( #6662 ), #10461, .T. ) ;
#11453=ADVANCED_FACE ( 'NONE', ( #8028 ), #1375, .F. ) ;
#11454=ORIENTED_EDGE ( 'NONE', *, *, #2944, .T. ) ;
#11458=DIRECTION ( 'NONE',  ( -1.000000000000000000, -3.903127820947815962E-18, 0.000000000000000000 ) ) ;
#11473=DIRECTION ( 'NONE',  ( -1.000000000000000000, 0.000000000000000000, 0.000000000000000000 ) ) ;
#11477=EDGE_CURVE ( 'NONE', #6450, #3193, #448, .T. ) ;
#11502=ADVANCED_FACE ( 'NONE', ( #5080 ), #507, .T. ) ;
#11525=EDGE_CURVE ( 'NONE', #10109, #3666, #2266, .T. ) ;
#11538=DIRECTION ( 'NONE',  ( 0.000000000000000000, 0.7900737791495477946, 0.6130117645692876316 ) ) ;
#11562=ORIENTED_EDGE ( 'NONE', *, *, #4166, .F. ) ;
#11569=EDGE_LOOP ( 'NONE', ( #6598, #12033, #3262, #6284 ) ) ;
#11575=FACE_OUTER_BOUND ( 'NONE', #12112, .T. ) ;
#11579=ORIENTED_EDGE ( 'NONE', *, *, #12100, .F. ) ;
#11586=VERTEX_POINT ( 'NONE', #1816 ) ;
#11604=VERTEX_POINT ( 'NONE', #10312 ) ;
#11605=EDGE_CURVE ( 'NONE', #7419, #6113, #8431, .T. ) ;
#11608=AXIS2_PLACEMENT_3D ( 'NONE', #2506, #6327, #9205 ) ;
#11645=ORIENTED_EDGE ( 'NONE', *, *, #6224, .F. ) ;
#11661=VERTEX_POINT ( 'NONE', #1695 ) ;
#11690=DIRECTION ( 'NONE',  ( -1.000000000000000000, 0.000000000000000000, 0.000000000000000000 ) ) ;
#11706=DIRECTION ( 'NONE',  ( 0.000000000000000000, -1.000000000000000000, 0.000000000000000000 ) ) ;
#11716=ORIENTED_EDGE ( 'NONE', *, *, #7478, .T. ) ;
#11723=EDGE_CURVE ( 'NONE', #7555, #4240, #7234, .T. ) ;
#11727=ORIENTED_EDGE ( 'NONE', *, *, #2399, .T. ) ;
#11739=AXIS2_PLACEMENT_3D ( 'NONE', #9268, #11178, #6448 ) ;
#11741=DIRECTION ( 'NONE',  ( 1.000000000000000000, -0.000000000000000000, -0.000000000000000000 ) ) ;
#11748=DIRECTION ( 'NONE',  ( -1.000000000000000000, -3.903127820947815962E-18, 0.000000000000000000 ) ) ;
#11753=VECTOR ( 'NONE', #4274, 1000.000000000000000 ) ;
#11763=DIRECTION ( 'NONE',  ( 0.000000000000000000, 0.5068368027542901055, -0.8620420264545163302 ) ) ;
#11788=CIRCLE ( 'NONE', #3222, 5.999999999999999112 ) ;
#11797=VERTEX_POINT ( 'NONE', #2813 ) ;
#11831=AXIS2_PLACEMENT_3D ( 'NONE', #11308, #2810, #7571 ) ;
#11871=LINE ( 'NONE', #371, #8064 ) ;
#11876=DIRECTION ( 'NONE',  ( -2.731402571913187487E-17, -0.5883347247165658933, 0.8086174940555531654 ) ) ;
#11881=EDGE_CURVE ( 'NONE', #6450, #10109, #436, .T. ) ;
#11885=LINE ( 'NONE', #2206, #172 ) ;
#11887=DIRECTION ( 'NONE',  ( -1.000000000000000000, -0.000000000000000000, -0.000000000000000000 ) ) ;
#11919=CARTESIAN_POINT ( 'NONE',  ( 37.00000000000000711, -2.263420294706660396, 4.458354917400590978 ) ) ;
#11925=DIRECTION ( 'NONE',  ( 0.000000000000000000, 0.8772744497699203059, 0.4799891038147465760 ) ) ;
#11945=VERTEX_POINT ( 'NONE', #9939 ) ;
#11954=MECHANICAL_DESIGN_GEOMETRIC_PRESENTATION_REPRESENTATION('',(#5777),#11362);
#11991=VECTOR ( 'NONE', #7177, 1000.000000000000000 ) ;
#11997=FILL_AREA_STYLE_COLOUR ( '', #9625 ) ;
#12005=AXIS2_PLACEMENT_3D ( 'NONE', #5915, #5717, #9536 ) ;
#12008=DIRECTION ( 'NONE',  ( 1.387778780781445984E-17, 0.7900737791495477946, 0.6130117645692875206 ) ) ;
#12018=ORIENTED_EDGE ( 'NONE', *, *, #8830, .F. ) ;
#12033=ORIENTED_EDGE ( 'NONE', *, *, #3699, .T. ) ;
#12058=DIRECTION ( 'NONE',  ( 0.000000000000000000, -1.000000000000000000, 0.000000000000000000 ) ) ;
#12078=DIRECTION ( 'NONE',  ( 0.000000000000000000, 0.7900737791495477946, 0.6130117645692876316 ) ) ;
#12081=CARTESIAN_POINT ( 'NONE',  ( 43.00000000000000000, 3.903127820947864496E-18, 0.000000000000000000 ) ) ;
#12082=PLANE ( 'NONE',  #4623 ) ;
#12091=ORIENTED_EDGE ( 'NONE', *, *, #8939, .T. ) ;
#12100=EDGE_CURVE ( 'NONE', #10112, #11945, #10034, .T. ) ;
#12101=DIRECTION ( 'NONE',  ( -1.000000000000000000, 0.000000000000000000, 0.000000000000000000 ) ) ;
#12104=EDGE_CURVE ( 'NONE', #11586, #9428, #7855, .T. ) ;
#12112=EDGE_LOOP ( 'NONE', ( #4543, #1611, #2643, #12211 ) ) ;
#12115=CARTESIAN_POINT ( 'NONE',  ( 36.00000000000000711, -4.104405154062230115E-16, -2.224720805914714718E-17 ) ) ;
#12122=ORIENTED_EDGE ( 'NONE', *, *, #11477, .T. ) ;
#12132=EDGE_LOOP ( 'NONE', ( #6724, #2682, #2305, #1495 ) ) ;
#12153=CARTESIAN_POINT ( 'NONE',  ( 37.00000000000000711, 0.000000000000000000, -1.500000000000000000 ) ) ;
#12158=ORIENTED_EDGE ( 'NONE', *, *, #4554, .T. ) ;
#12182=CYLINDRICAL_SURFACE ( 'NONE', #2840, 5.000000000000000000 ) ;
#12211=ORIENTED_EDGE ( 'NONE', *, *, #4117, .T. ) ;
#12223=CARTESIAN_POINT ( 'NONE',  ( 36.00000000000000711, -2.263420294706660396, 4.458354917400590978 ) ) ;
#12225=DIRECTION ( 'NONE',  ( 0.000000000000000000, 1.000000000000000000, -0.000000000000000000 ) ) ;
#12236=EDGE_CURVE ( 'NONE', #11797, #3600, #6417, .T. ) ;
#12244=( NAMED_UNIT ( * ) SI_UNIT ( $, .STERADIAN. ) SOLID_ANGLE_UNIT ( ) );
#12248=ORIENTED_EDGE ( 'NONE', *, *, #7478, .F. ) ;
#12265=EDGE_CURVE ( 'NONE', #11945, #7392, #10226, .T. ) ;
#12276=DIRECTION ( 'NONE',  ( 0.000000000000000000, -0.4526840589413320126, 0.8916709834801178625 ) ) ;
#12281=ORIENTED_EDGE ( 'NONE', *, *, #10127, .F. ) ;
#12308=CARTESIAN_POINT ( 'NONE',  ( -36.00000000000000000, 7.347880794884118750E-16, 5.999999999999999112 ) ) ;
#12314=CARTESIAN_POINT ( 'NONE',  ( 45.00000000000000000, 0.000000000000000000, 0.000000000000000000 ) ) ;
#12333=CARTESIAN_POINT ( 'NONE',  ( 37.00000000000000711, 4.769696007084728073, -1.500000000000000444 ) ) ;
#12339=CIRCLE ( 'NONE', #11739, 4.799999999999999822 ) ;
#12344=PLANE ( 'NONE',  #1621 ) ;
#12406=COLOUR_RGB('Off White',0.89,0.88,0.83);
#12407=FILL_AREA_STYLE_COLOUR('',#12406);
#12408=FILL_AREA_STYLE('',(#12407));
#12409=SURFACE_STYLE_FILL_AREA(#12408);
#12410=SURFACE_SIDE_STYLE('',(#12409));
#12411=SURFACE_STYLE_USAGE(.BOTH.,#12410);
#12412=PRESENTATION_STYLE_ASSIGNMENT((#12411));
ENDSEC;
END-ISO-10303-21;
